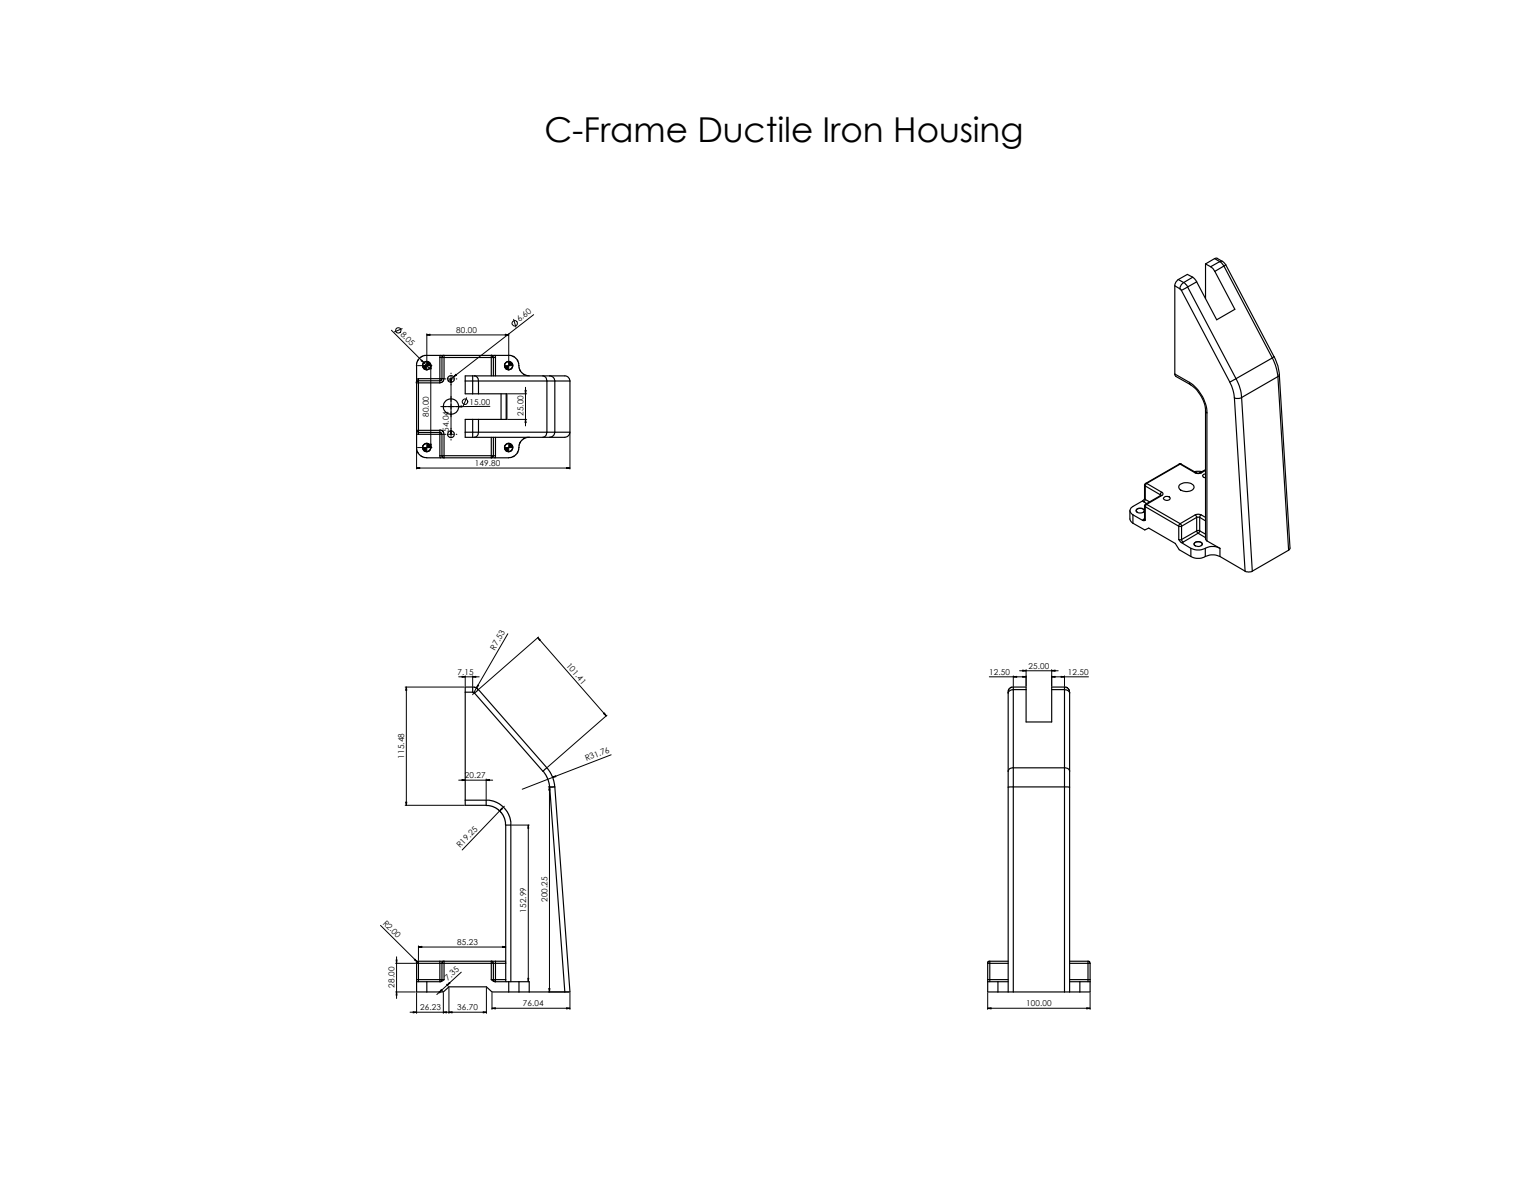
ISO-10303-21;
HEADER;
FILE_DESCRIPTION (('STEP AP214'),
    '1' );
FILE_NAME ('C-Frame Ductile Iron Housing.step',
    '2026-10-20T14:49:59',
    ( '' ),
    ( '' ),
    'SwSTEP 2.0',
    'SolidWorks 2025',
    '' );
FILE_SCHEMA (( 'AUTOMOTIVE_DESIGN' ));
ENDSEC;

DATA;
#1=AXIS2_PLACEMENT_3D ( 'NONE', #1947, #6240, #1422 ) ;
#5=( BOUNDED_CURVE ( )  B_SPLINE_CURVE ( 3, ( #4259, #2824, #7496, #242 ),
 .UNSPECIFIED., .F., .F. ) 
 B_SPLINE_CURVE_WITH_KNOTS ( ( 4, 4 ),
 ( 3.228493165690314637, 4.434806757669079502 ),
 .UNSPECIFIED. ) 
 CURVE ( )  GEOMETRIC_REPRESENTATION_ITEM ( )  RATIONAL_B_SPLINE_CURVE ( ( 1.000000000000000000, 0.8823660295963204891, 0.8823660295963204891, 1.000000000000000000 ) ) 
 REPRESENTATION_ITEM ( '' )  );
#7=EDGE_CURVE ( 'NONE', #389, #4565, #2197, .T. ) ;
#8=VERTEX_POINT ( 'NONE', #6223 ) ;
#15=ORIENTED_EDGE ( 'NONE', *, *, #8479, .F. ) ;
#18=ORIENTED_EDGE ( 'NONE', *, *, #2489, .T. ) ;
#21=DIRECTION ( 'NONE',  ( -1.000000000000000000, 0.000000000000000000, -1.396588258780021135E-16 ) ) ;
#25=DIRECTION ( 'NONE',  ( -1.000000000000000000, 0.000000000000000000, 0.000000000000000000 ) ) ;
#30=ADVANCED_FACE ( 'NONE', ( #9249 ), #6112, .F. ) ;
#31=EDGE_CURVE ( 'NONE', #2894, #7105, #9463, .T. ) ;
#36=VERTEX_POINT ( 'NONE', #6165 ) ;
#37=CIRCLE ( 'NONE', #7311, 10.00000000000000178 ) ;
#40=CARTESIAN_POINT ( 'NONE',  ( 2.108096605167895612E-14, -117.1457019118819005, -25.15769640663941686 ) ) ;
#42=CARTESIAN_POINT ( 'NONE',  ( 39.99999999999998579, -135.1707019118818778, -36.00000000000002842 ) ) ;
#43=DIRECTION ( 'NONE',  ( -1.000000000000000000, 0.000000000000000000, 0.000000000000000000 ) ) ;
#44=LINE ( 'NONE', #8251, #3603 ) ;
#45=VECTOR ( 'NONE', #8925, 1000.000000000000000 ) ;
#46=EDGE_CURVE ( 'NONE', #9808, #836, #8928, .T. ) ;
#47=VERTEX_POINT ( 'NONE', #6006 ) ;
#48=CARTESIAN_POINT ( 'NONE',  ( -16.29350689640809691, -186.9457019118818835, 23.72119897386845722 ) ) ;
#49=ORIENTED_EDGE ( 'NONE', *, *, #1262, .T. ) ;
#55=DIRECTION ( 'NONE',  ( -0.7367503238654704578, -0.6761648913424330720, -0.000000000000000000 ) ) ;
#56=CARTESIAN_POINT ( 'NONE',  ( 99.80027788547049283, -145.1457019118819574, 25.00000000000000000 ) ) ;
#57=LINE ( 'NONE', #8266, #434 ) ;
#58=ORIENTED_EDGE ( 'NONE', *, *, #5513, .T. ) ;
#59=VERTEX_POINT ( 'NONE', #6862 ) ;
#64=ADVANCED_FACE ( 'NONE', ( #10099 ), #3860, .F. ) ;
#65=DIRECTION ( 'NONE',  ( -0.000000000000000000, -0.000000000000000000, -1.000000000000000000 ) ) ;
#69=ORIENTED_EDGE ( 'NONE', *, *, #7396, .F. ) ;
#70=FACE_OUTER_BOUND ( 'NONE', #3100, .T. ) ;
#71=VECTOR ( 'NONE', #3438, 1000.000000000000000 ) ;
#73=CIRCLE ( 'NONE', #8358, 4.025000000000000355 ) ;
#74=ORIENTED_EDGE ( 'NONE', *, *, #80, .F. ) ;
#75=UNCERTAINTY_MEASURE_WITH_UNIT (LENGTH_MEASURE( 1.000000000000000082E-05 ), #6894, 'distance_accuracy_value', 'NONE');
#76=ORIENTED_EDGE ( 'NONE', *, *, #6234, .T. ) ;
#79=LINE ( 'NONE', #3304, #8495 ) ;
#80=EDGE_CURVE ( 'NONE', #1253, #6094, #1141, .T. ) ;
#81=DIRECTION ( 'NONE',  ( 0.000000000000000000, 1.000000000000000000, 0.000000000000000000 ) ) ;
#82=LINE ( 'NONE', #7283, #1628 ) ;
#86=VERTEX_POINT ( 'NONE', #4732 ) ;
#87=CARTESIAN_POINT ( 'NONE',  ( 37.22511195853866894, 17.84145331825995484, -25.00000000000000355 ) ) ;
#92=AXIS2_PLACEMENT_3D ( 'NONE', #1690, #1849, #8953 ) ;
#93=DIRECTION ( 'NONE',  ( 0.000000000000000000, -0.000000000000000000, -1.000000000000000000 ) ) ;
#98=LINE ( 'NONE', #6716, #4014 ) ;
#102=CYLINDRICAL_SURFACE ( 'NONE', #1212, 2.000000000000001776 ) ;
#103=EDGE_CURVE ( 'NONE', #7113, #7038, #645, .T. ) ;
#108=DIRECTION ( 'NONE',  ( 1.000000000000000000, 0.000000000000000000, 0.000000000000000000 ) ) ;
#109=VERTEX_POINT ( 'NONE', #7181 ) ;
#110=ORIENTED_EDGE ( 'NONE', *, *, #8315, .T. ) ;
#111=ORIENTED_EDGE ( 'NONE', *, *, #371, .T. ) ;
#114=ORIENTED_EDGE ( 'NONE', *, *, #3993, .T. ) ;
#115=ORIENTED_EDGE ( 'NONE', *, *, #7748, .F. ) ;
#116=DIRECTION ( 'NONE',  ( 0.000000000000000000, 0.000000000000000000, 1.000000000000000000 ) ) ;
#118=EDGE_CURVE ( 'NONE', #991, #7873, #6383, .T. ) ;
#119=DIRECTION ( 'NONE',  ( -0.000000000000000000, 1.000000000000000000, -0.000000000000000000 ) ) ;
#120=DIRECTION ( 'NONE',  ( -0.000000000000000000, 1.000000000000000000, -0.000000000000000000 ) ) ;
#123=DIRECTION ( 'NONE',  ( -0.000000000000000000, 1.000000000000000000, -0.000000000000000000 ) ) ;
#126=VECTOR ( 'NONE', #3375, 1000.000000000000000 ) ;
#127=CARTESIAN_POINT ( 'NONE',  ( 39.99999999999998579, -115.1457019118818863, -50.00000000000002132 ) ) ;
#128=EDGE_CURVE ( 'NONE', #9477, #9534, #1310, .T. ) ;
#129=VECTOR ( 'NONE', #2614, 1000.000000000000000 ) ;
#130=ORIENTED_EDGE ( 'NONE', *, *, #2088, .F. ) ;
#135=DIRECTION ( 'NONE',  ( 0.000000000000000000, 0.000000000000000000, -1.000000000000000000 ) ) ;
#137=DIRECTION ( 'NONE',  ( 0.000000000000000000, 0.000000000000000000, 1.000000000000000000 ) ) ;
#139=VECTOR ( 'NONE', #10142, 1000.000000000000000 ) ;
#142=EDGE_CURVE ( 'NONE', #5755, #3381, #6273, .T. ) ;
#143=ORIENTED_EDGE ( 'NONE', *, *, #3330, .T. ) ;
#144=DIRECTION ( 'NONE',  ( -1.000000000000000000, 0.000000000000000000, 0.000000000000000000 ) ) ;
#145=ORIENTED_EDGE ( 'NONE', *, *, #5104, .T. ) ;
#149=AXIS2_PLACEMENT_3D ( 'NONE', #5640, #2363, #7980 ) ;
#150=FACE_BOUND ( 'NONE', #8598, .T. ) ;
#151=FACE_OUTER_BOUND ( 'NONE', #4068, .T. ) ;
#159=ORIENTED_EDGE ( 'NONE', *, *, #5597, .F. ) ;
#160=CARTESIAN_POINT ( 'NONE',  ( -2.293506896408097795, 120.5696653505793705, 16.00000000000000711 ) ) ;
#161=FACE_OUTER_BOUND ( 'NONE', #8002, .T. ) ;
#162=DIRECTION ( 'NONE',  ( 0.000000000000000000, 0.000000000000000000, -1.000000000000000000 ) ) ;
#163=CARTESIAN_POINT ( 'NONE',  ( 0.000000000000000000, -135.1457019118818721, 49.99999999999997868 ) ) ;
#164=DIRECTION ( 'NONE',  ( -0.000000000000000000, 1.000000000000000000, -0.000000000000000000 ) ) ;
#165=DIRECTION ( 'NONE',  ( 1.000000000000000000, 0.000000000000000000, -0.000000000000000000 ) ) ;
#170=EDGE_LOOP ( 'NONE', ( #1521, #9934, #3722, #2301 ) ) ;
#172=VERTEX_POINT ( 'NONE', #5530 ) ;
#174=CARTESIAN_POINT ( 'NONE',  ( 4.856471286862176662, 145.0444252872335937, -25.00000000000000355 ) ) ;
#175=CARTESIAN_POINT ( 'NONE',  ( 39.99999999999998579, -135.1707019118818778, -40.00000000000002132 ) ) ;
#176=ORIENTED_EDGE ( 'NONE', *, *, #2184, .F. ) ;
#178=ORIENTED_EDGE ( 'NONE', *, *, #10204, .T. ) ;
#180=ADVANCED_FACE ( 'NONE', ( #7280 ), #10317, .T. ) ;
#181=ORIENTED_EDGE ( 'NONE', *, *, #259, .T. ) ;
#184=DIRECTION ( 'NONE',  ( 0.6761648913424331830, 0.7367503238654705688, 0.000000000000000000 ) ) ;
#185=FACE_OUTER_BOUND ( 'NONE', #1495, .T. ) ;
#189=ORIENTED_EDGE ( 'NONE', *, *, #3670, .T. ) ;
#192=PRODUCT_CONTEXT ( 'NONE', #5163, 'mechanical' ) ;
#193=ORIENTED_EDGE ( 'NONE', *, *, #118, .T. ) ;
#194=CARTESIAN_POINT ( 'NONE',  ( 0.000000000000000000, -135.1457019118818721, 0.000000000000000000 ) ) ;
#196=ADVANCED_FACE ( 'NONE', ( #3094 ), #2303, .F. ) ;
#201=DIRECTION ( 'NONE',  ( -0.000000000000000000, 1.000000000000000000, -0.000000000000000000 ) ) ;
#204=AXIS2_PLACEMENT_3D ( 'NONE', #9863, #838, #6454 ) ;
#206=CIRCLE ( 'NONE', #9340, 5.000000000000000888 ) ;
#207=EDGE_LOOP ( 'NONE', ( #1735, #9870, #2298, #4217 ) ) ;
#208=DIRECTION ( 'NONE',  ( -0.000000000000000000, -0.000000000000000000, -1.000000000000000000 ) ) ;
#210=DIRECTION ( 'NONE',  ( 0.000000000000000000, -1.000000000000000000, 0.000000000000000000 ) ) ;
#211=DIRECTION ( 'NONE',  ( 1.000000000000000000, 0.000000000000000000, 0.000000000000000000 ) ) ;
#215=CARTESIAN_POINT ( 'NONE',  ( 39.99999999999997158, -135.1707019118818778, 35.99999999999998579 ) ) ;
#216=ORIENTED_EDGE ( 'NONE', *, *, #1932, .F. ) ;
#219=ORIENTED_EDGE ( 'NONE', *, *, #8508, .T. ) ;
#220=CIRCLE ( 'NONE', #5954, 2.000000000000001776 ) ;
#222=DIRECTION ( 'NONE',  ( 1.000000000000000000, -0.000000000000000000, -0.000000000000000000 ) ) ;
#223=ADVANCED_FACE ( 'NONE', ( #968 ), #9262, .F. ) ;
#225=EDGE_CURVE ( 'NONE', #5542, #7357, #9074, .T. ) ;
#226=ORIENTED_EDGE ( 'NONE', *, *, #6379, .T. ) ;
#227=CARTESIAN_POINT ( 'NONE',  ( 14.70649310359190309, 120.5696653505793705, 20.00000000000000711 ) ) ;
#228=TOROIDAL_SURFACE ( 'NONE', #6479, 2.525240063345735475, 5.000000000000000000 ) ;
#230=CARTESIAN_POINT ( 'NONE',  ( 14.70649310359190309, 120.5696653505793705, 20.00000000000000711 ) ) ;
#232=ORIENTED_EDGE ( 'NONE', *, *, #10101, .T. ) ;
#234=CARTESIAN_POINT ( 'NONE',  ( -40.00000000000001421, -145.1457019118819005, -40.00000000000002132 ) ) ;
#235=VECTOR ( 'NONE', #6566, 1000.000000000000000 ) ;
#239=EDGE_CURVE ( 'NONE', #4318, #3843, #3408, .T. ) ;
#242=CARTESIAN_POINT ( 'NONE',  ( -18.34874108452141783, -140.1746510883711778, 7.212905963064383918 ) ) ;
#243=ORIENTED_EDGE ( 'NONE', *, *, #6508, .F. ) ;
#244=CARTESIAN_POINT ( 'NONE',  ( -40.00000000000002842, -135.1457019118818721, 39.99999999999997868 ) ) ;
#246=ORIENTED_EDGE ( 'NONE', *, *, #9487, .F. ) ;
#248=LINE ( 'NONE', #2462, #7946 ) ;
#249=VERTEX_POINT ( 'NONE', #5785 ) ;
#251=EDGE_CURVE ( 'NONE', #7304, #5030, #3169, .T. ) ;
#252=FACE_BOUND ( 'NONE', #5488, .T. ) ;
#253=CARTESIAN_POINT ( 'NONE',  ( -50.00000000000002132, -115.1457019118818863, 23.15769640663938134 ) ) ;
#256=DIRECTION ( 'NONE',  ( 0.000000000000000000, 0.000000000000000000, -1.000000000000000000 ) ) ;
#257=CARTESIAN_POINT ( 'NONE',  ( -23.15769640663940976, -133.1457019118818721, 49.99999999999997868 ) ) ;
#259=EDGE_CURVE ( 'NONE', #9948, #541, #8974, .T. ) ;
#260=EDGE_LOOP ( 'NONE', ( #7752, #8876, #7839, #4575 ) ) ;
#261=AXIS2_PLACEMENT_3D ( 'NONE', #3282, #9005, #108 ) ;
#262=DIRECTION ( 'NONE',  ( 1.000000000000000000, 0.000000000000000000, 0.000000000000000000 ) ) ;
#265=FACE_OUTER_BOUND ( 'NONE', #5639, .T. ) ;
#266=DIRECTION ( 'NONE',  ( -0.000000000000000000, 1.000000000000000000, -0.000000000000000000 ) ) ;
#267=B_SPLINE_CURVE_WITH_KNOTS ( 'NONE', 3,
 ( #1751, #6037, #5296, #7584 ),
 .UNSPECIFIED., .F., .F.,
 ( 4, 4 ),
 ( 0.000000000000000000, 0.0007942240325546930492 ),
 .UNSPECIFIED. ) ;
#269=DIRECTION ( 'NONE',  ( 0.000000000000000000, 0.000000000000000000, -1.000000000000000000 ) ) ;
#271=CIRCLE ( 'NONE', #8898, 4.999999999999997335 ) ;
#273=ORIENTED_EDGE ( 'NONE', *, *, #8937, .T. ) ;
#275=ORIENTED_EDGE ( 'NONE', *, *, #9151, .T. ) ;
#280=ORIENTED_EDGE ( 'NONE', *, *, #3281, .F. ) ;
#282=AXIS2_PLACEMENT_3D ( 'NONE', #1944, #4741, #724 ) ;
#284=CYLINDRICAL_SURFACE ( 'NONE', #9989, 2.000000000000001776 ) ;
#285=CIRCLE ( 'NONE', #7057, 3.999999999999996447 ) ;
#287=EDGE_CURVE ( 'NONE', #249, #2514, #5099, .T. ) ;
#293=CARTESIAN_POINT ( 'NONE',  ( -48.00000000000002132, -133.1457019118818721, -27.15769640663945594 ) ) ;
#296=DIRECTION ( 'NONE',  ( -0.000000000000000000, 1.000000000000000000, -0.000000000000000000 ) ) ;
#297=CARTESIAN_POINT ( 'NONE',  ( 39.99999999999997158, -135.1457019118818721, 39.99999999999997868 ) ) ;
#298=ORIENTED_EDGE ( 'NONE', *, *, #6850, .F. ) ;
#301=ORIENTED_EDGE ( 'NONE', *, *, #542, .F. ) ;
#305=AXIS2_PLACEMENT_3D ( 'NONE', #4703, #7939, #5550 ) ;
#309=DIRECTION ( 'NONE',  ( -0.000000000000000000, -0.000000000000000000, 1.000000000000000000 ) ) ;
#311=EDGE_LOOP ( 'NONE', ( #929, #9154, #4963 ) ) ;
#312=AXIS2_PLACEMENT_3D ( 'NONE', #483, #2971, #4458 ) ;
#313=CARTESIAN_POINT ( 'NONE',  ( 53.40242741783141156, 42.08684478514406635, -30.00000000000000355 ) ) ;
#319=ORIENTED_EDGE ( 'NONE', *, *, #618, .T. ) ;
#320=DIRECTION ( 'NONE',  ( -1.387778780781445676E-16, 0.000000000000000000, 1.000000000000000000 ) ) ;
#321=DIRECTION ( 'NONE',  ( 0.000000000000000000, 0.000000000000000000, 1.000000000000000000 ) ) ;
#323=CARTESIAN_POINT ( 'NONE',  ( -38.19229777560033057, 37.08684478514405214, -12.50000000000000000 ) ) ;
#327=ORIENTED_EDGE ( 'NONE', *, *, #7111, .T. ) ;
#329=CARTESIAN_POINT ( 'NONE',  ( 14.70649310359190309, 120.5696653505793705, -20.00000000000000711 ) ) ;
#330=CIRCLE ( 'NONE', #4045, 4.000000000000000000 ) ;
#332=EDGE_CURVE ( 'NONE', #8658, #7935, #9280, .T. ) ;
#335=DIRECTION ( 'NONE',  ( 0.000000000000000000, 0.000000000000000000, 1.000000000000000000 ) ) ;
#336=ORIENTED_EDGE ( 'NONE', *, *, #3079, .T. ) ;
#337=CARTESIAN_POINT ( 'NONE',  ( 14.70649310359190309, 80.56966535057935630, -20.00000000000000711 ) ) ;
#340=ORIENTED_EDGE ( 'NONE', *, *, #1843, .F. ) ;
#346=CARTESIAN_POINT ( 'NONE',  ( 37.22797271129282848, -133.4137847133962396, -25.17122046401099311 ) ) ;
#348=DIRECTION ( 'NONE',  ( 0.000000000000000000, 1.000000000000000000, -0.000000000000000000 ) ) ;
#349=ORIENTED_EDGE ( 'NONE', *, *, #1530, .T. ) ;
#351=CARTESIAN_POINT ( 'NONE',  ( 39.99999999999998579, -135.1457019118818721, -40.00000000000002132 ) ) ;
#352=DIRECTION ( 'NONE',  ( 0.000000000000000000, 0.000000000000000000, 1.000000000000000000 ) ) ;
#359=ORIENTED_EDGE ( 'NONE', *, *, #6276, .F. ) ;
#366=ORIENTED_EDGE ( 'NONE', *, *, #3251, .T. ) ;
#371=EDGE_CURVE ( 'NONE', #6079, #5542, #9235, .T. ) ;
#373=EDGE_CURVE ( 'NONE', #3710, #6945, #2925, .T. ) ;
#375=ORIENTED_EDGE ( 'NONE', *, *, #6294, .F. ) ;
#377=ORIENTED_EDGE ( 'NONE', *, *, #2708, .T. ) ;
#381=LINE ( 'NONE', #2917, #3516 ) ;
#385=AXIS2_PLACEMENT_3D ( 'NONE', #470, #266, #3704 ) ;
#388=ORIENTED_EDGE ( 'NONE', *, *, #4709, .T. ) ;
#389=VERTEX_POINT ( 'NONE', #6099 ) ;
#391=LINE ( 'NONE', #7015, #708 ) ;
#392=DIRECTION ( 'NONE',  ( -0.7525569905852185215, -0.6585271261848818503, 0.000000000000000000 ) ) ;
#400=CARTESIAN_POINT ( 'NONE',  ( 99.80027788547049283, -145.1457019118819005, 25.00000000000000000 ) ) ;
#403=LINE ( 'NONE', #4479, #10289 ) ;
#406=AXIS2_PLACEMENT_3D ( 'NONE', #8418, #9973, #3651 ) ;
#408=CARTESIAN_POINT ( 'NONE',  ( -16.29350689640809691, -140.1746510883711778, -27.01918567566963247 ) ) ;
#412=EDGE_LOOP ( 'NONE', ( #6955, #1615, #901, #8803 ) ) ;
#413=CARTESIAN_POINT ( 'NONE',  ( 39.99999999999997158, -145.1457019118819005, 43.99999999999997158 ) ) ;
#414=EDGE_CURVE ( 'NONE', #7304, #3508, #5358, .T. ) ;
#415=VERTEX_POINT ( 'NONE', #7799 ) ;
#416=AXIS2_PLACEMENT_3D ( 'NONE', #6605, #8136, #2577 ) ;
#421=FACE_OUTER_BOUND ( 'NONE', #4486, .T. ) ;
#424=VECTOR ( 'NONE', #10366, 1000.000000000000000 ) ;
#425=ORIENTED_EDGE ( 'NONE', *, *, #4709, .F. ) ;
#426=VERTEX_POINT ( 'NONE', #6154 ) ;
#427=CARTESIAN_POINT ( 'NONE',  ( 39.99999999999998579, -135.1457019118818721, -40.00000000000002132 ) ) ;
#429=EDGE_CURVE ( 'NONE', #10221, #9616, #9343, .T. ) ;
#433=DIRECTION ( 'NONE',  ( 0.000000000000000000, 0.000000000000000000, 1.000000000000000000 ) ) ;
#434=VECTOR ( 'NONE', #2697, 1000.000000000000000 ) ;
#436=CARTESIAN_POINT ( 'NONE',  ( 39.99999999999998579, -135.1457019118818721, -44.02500000000001990 ) ) ;
#437=CIRCLE ( 'NONE', #6179, 10.00000000000000178 ) ;
#440=ORIENTED_EDGE ( 'NONE', *, *, #2696, .F. ) ;
#446=CYLINDRICAL_SURFACE ( 'NONE', #9247, 1.999999999999998224 ) ;
#448=FACE_OUTER_BOUND ( 'NONE', #668, .T. ) ;
#449=AXIS2_PLACEMENT_3D ( 'NONE', #1185, #3570, #1133 ) ;
#451=DIRECTION ( 'NONE',  ( 1.000000000000000000, 0.000000000000000000, -0.000000000000000000 ) ) ;
#453=DIRECTION ( 'NONE',  ( 8.379529552680108569E-16, 0.000000000000000000, -1.000000000000000000 ) ) ;
#454=ORIENTED_EDGE ( 'NONE', *, *, #516, .F. ) ;
#456=CARTESIAN_POINT ( 'NONE',  ( 23.15769640663935292, -117.1457019118819005, 2.263923683133336310E-14 ) ) ;
#457=EDGE_CURVE ( 'NONE', #10082, #9303, #1997, .T. ) ;
#461=ORIENTED_EDGE ( 'NONE', *, *, #1064, .F. ) ;
#462=CARTESIAN_POINT ( 'NONE',  ( 0.000000000000000000, -135.1457019118818721, -30.00000000000000355 ) ) ;
#463=AXIS2_PLACEMENT_3D ( 'NONE', #984, #7454, #8830 ) ;
#464=ORIENTED_EDGE ( 'NONE', *, *, #46, .F. ) ;
#465=CARTESIAN_POINT ( 'NONE',  ( -23.15769640663937423, -117.1457019118819005, -50.00000000000002132 ) ) ;
#470=CARTESIAN_POINT ( 'NONE',  ( 39.99999999999997158, -135.1457019118818721, 39.99999999999997868 ) ) ;
#473=DIRECTION ( 'NONE',  ( -0.000000000000000000, -1.000000000000000000, -0.000000000000000000 ) ) ;
#475=EDGE_CURVE ( 'NONE', #3710, #4318, #8599, .T. ) ;
#478=CARTESIAN_POINT ( 'NONE',  ( -2.293506896408094242, 152.5696653505793279, -12.50000000000000000 ) ) ;
#480=CARTESIAN_POINT ( 'NONE',  ( 14.70649310359190309, 120.5696653505793705, 20.00000000000000711 ) ) ;
#482=CARTESIAN_POINT ( 'NONE',  ( 38.19229777560031636, 118.3760186273086816, -12.50000000000000000 ) ) ;
#483=CARTESIAN_POINT ( 'NONE',  ( 0.000000000000000000, -115.1457019118818863, -50.00000000000002132 ) ) ;
#485=AXIS2_PLACEMENT_3D ( 'NONE', #1777, #6653, #7502 ) ;
#492=ORIENTED_EDGE ( 'NONE', *, *, #6447, .F. ) ;
#496=DIRECTION ( 'NONE',  ( 0.000000000000000000, 1.000000000000000000, 0.000000000000000000 ) ) ;
#499=LINE ( 'NONE', #10311, #7721 ) ;
#500=EDGE_CURVE ( 'NONE', #47, #3843, #7698, .T. ) ;
#505=CARTESIAN_POINT ( 'NONE',  ( 25.15769640663936002, -115.1457019118818863, -3.513494341946486113E-15 ) ) ;
#507=DIRECTION ( 'NONE',  ( -1.000000000000000000, 0.000000000000000000, 0.000000000000000000 ) ) ;
#508=DIRECTION ( 'NONE',  ( -0.000000000000000000, 1.000000000000000000, -0.000000000000000000 ) ) ;
#511=CYLINDRICAL_SURFACE ( 'NONE', #5792, 4.999999999999997335 ) ;
#514=LINE ( 'NONE', #8516, #2322 ) ;
#515=ORIENTED_EDGE ( 'NONE', *, *, #6735, .T. ) ;
#516=EDGE_CURVE ( 'NONE', #9939, #3381, #7904, .T. ) ;
#520=( LENGTH_UNIT ( ) NAMED_UNIT ( * ) SI_UNIT ( .MILLI., .METRE. ) );
#521=DIRECTION ( 'NONE',  ( 0.000000000000000000, -1.000000000000000000, 0.000000000000000000 ) ) ;
#523=DIRECTION ( 'NONE',  ( 0.000000000000000000, 1.000000000000000000, -0.000000000000000000 ) ) ;
#527=AXIS2_PLACEMENT_3D ( 'NONE', #7457, #1037, #6552 ) ;
#528=ORIENTED_EDGE ( 'NONE', *, *, #8703, .F. ) ;
#529=ADVANCED_FACE ( 'NONE', ( #748 ), #598, .F. ) ;
#530=DIRECTION ( 'NONE',  ( -1.387778780781445676E-16, 0.000000000000000000, 1.000000000000000000 ) ) ;
#531=CARTESIAN_POINT ( 'NONE',  ( -2.293506896408097795, 152.5696653505793279, 30.00000000000000355 ) ) ;
#533=LINE ( 'NONE', #2178, #8761 ) ;
#535=VECTOR ( 'NONE', #5204, 1000.000000000000227 ) ;
#538=AXIS2_PLACEMENT_3D ( 'NONE', #3174, #3070, #8843 ) ;
#539=ORIENTED_EDGE ( 'NONE', *, *, #7426, .F. ) ;
#540=AXIS2_PLACEMENT_3D ( 'NONE', #9014, #1857, #5669 ) ;
#541=VERTEX_POINT ( 'NONE', #3185 ) ;
#542=EDGE_CURVE ( 'NONE', #1314, #8114, #798, .T. ) ;
#546=FACE_OUTER_BOUND ( 'NONE', #2266, .T. ) ;
#547=DIRECTION ( 'NONE',  ( -0.000000000000000000, 1.000000000000000000, -0.000000000000000000 ) ) ;
#548=DIRECTION ( 'NONE',  ( 0.000000000000000000, -0.000000000000000000, -1.000000000000000000 ) ) ;
#549=AXIS2_PLACEMENT_3D ( 'NONE', #9186, #9892, #1766 ) ;
#550=ORIENTED_EDGE ( 'NONE', *, *, #3594, .F. ) ;
#552=CARTESIAN_POINT ( 'NONE',  ( -48.00000000000002132, -117.1457019118819005, -25.15769640663945950 ) ) ;
#553=DIRECTION ( 'NONE',  ( 1.000000000000000000, 0.000000000000000000, 0.000000000000000000 ) ) ;
#554=EDGE_CURVE ( 'NONE', #10372, #47, #7122, .T. ) ;
#555=ORIENTED_EDGE ( 'NONE', *, *, #457, .T. ) ;
#557=CIRCLE ( 'NONE', #1228, 2.000000000000001776 ) ;
#560=CARTESIAN_POINT ( 'NONE',  ( 25.93999053166053415, -135.0799163051958942, -50.00000000000002132 ) ) ;
#561=CARTESIAN_POINT ( 'NONE',  ( -50.00000000000001421, -145.1457019118819005, -40.00000000000002132 ) ) ;
#563=DIRECTION ( 'NONE',  ( -1.000000000000000000, 0.000000000000000000, 0.000000000000000000 ) ) ;
#564=AXIS2_PLACEMENT_3D ( 'NONE', #9552, #1379, #738 ) ;
#568=CARTESIAN_POINT ( 'NONE',  ( -40.00000000000002842, -135.1457019118818721, 39.99999999999997868 ) ) ;
#569=ORIENTED_EDGE ( 'NONE', *, *, #2486, .T. ) ;
#570=ADVANCED_FACE ( 'NONE', ( #6415 ), #698, .F. ) ;
#573=DIRECTION ( 'NONE',  ( 0.000000000000000000, 1.000000000000000000, 0.000000000000000000 ) ) ;
#574=AXIS2_PLACEMENT_3D ( 'NONE', #10123, #6882, #3549 ) ;
#575=LINE ( 'NONE', #9043, #126 ) ;
#578=FACE_BOUND ( 'NONE', #834, .T. ) ;
#580=ADVANCED_FACE ( 'NONE', ( #5467, #8756 ), #7961, .F. ) ;
#581=VERTEX_POINT ( 'NONE', #8700 ) ;
#583=DIRECTION ( 'NONE',  ( 0.000000000000000000, 0.000000000000000000, -1.000000000000000000 ) ) ;
#586=CARTESIAN_POINT ( 'NONE',  ( -48.00000000000002132, -117.1457019118819005, -23.15769640663945594 ) ) ;
#587=DIRECTION ( 'NONE',  ( -0.000000000000000000, 0.000000000000000000, -1.000000000000000000 ) ) ;
#589=CARTESIAN_POINT ( 'NONE',  ( 14.70649310359190309, 120.5696653505793705, -20.00000000000000711 ) ) ;
#595=CIRCLE ( 'NONE', #4810, 2.000000000000001776 ) ;
#598=PLANE ( 'NONE',  #1493 ) ;
#599=CARTESIAN_POINT ( 'NONE',  ( 42.22511195853869026, -135.1457019118818721, -25.00000000000000355 ) ) ;
#602=DIRECTION ( 'NONE',  ( -0.000000000000000000, 1.000000000000000000, -0.000000000000000000 ) ) ;
#609=AXIS2_PLACEMENT_3D ( 'NONE', #4481, #3581, #5958 ) ;
#611=CARTESIAN_POINT ( 'NONE',  ( 25.28853996896956247, -134.8487302617674857, -50.00000000000001421 ) ) ;
#612=DIRECTION ( 'NONE',  ( 1.000000000000000000, 0.000000000000000000, 1.387778780781445676E-16 ) ) ;
#616=ADVANCED_FACE ( 'NONE', ( #8805 ), #1548, .T. ) ;
#618=EDGE_CURVE ( 'NONE', #5017, #8294, #9061, .T. ) ;
#619=ORIENTED_EDGE ( 'NONE', *, *, #4744, .F. ) ;
#620=CIRCLE ( 'NONE', #8401, 2.000000000000001776 ) ;
#626=CIRCLE ( 'NONE', #3497, 2.000000000000001776 ) ;
#627=DIRECTION ( 'NONE',  ( -0.000000000000000000, 1.000000000000000000, -0.000000000000000000 ) ) ;
#628=CARTESIAN_POINT ( 'NONE',  ( 39.99999999999998579, -135.1457019118818721, -40.00000000000002132 ) ) ;
#629=DIRECTION ( 'NONE',  ( -0.000000000000000000, 1.000000000000000000, -0.000000000000000000 ) ) ;
#631=PLANE ( 'NONE',  #5090 ) ;
#635=ORIENTED_EDGE ( 'NONE', *, *, #3138, .T. ) ;
#636=VECTOR ( 'NONE', #2330, 1000.000000000000000 ) ;
#637=CARTESIAN_POINT ( 'NONE',  ( 4.856471286862175774, 152.5696653505793279, -25.00000000000000355 ) ) ;
#638=ADVANCED_BREP_SHAPE_REPRESENTATION ( '', ( #3440, #4601 ), #9171 ) ;
#639=VECTOR ( 'NONE', #7530, 1000.000000000000000 ) ;
#640=VERTEX_POINT ( 'NONE', #4082 ) ;
#641=CARTESIAN_POINT ( 'NONE',  ( -16.29350689640809691, -140.1746510883711778, 0.000000000000000000 ) ) ;
#643=FACE_OUTER_BOUND ( 'NONE', #4818, .T. ) ;
#644=FACE_OUTER_BOUND ( 'NONE', #7569, .T. ) ;
#645=CIRCLE ( 'NONE', #4022, 2.000000000000001776 ) ;
#648=ORIENTED_EDGE ( 'NONE', *, *, #9261, .F. ) ;
#649=ORIENTED_EDGE ( 'NONE', *, *, #8829, .F. ) ;
#650=CIRCLE ( 'NONE', #9099, 5.000000000000000888 ) ;
#653=ORIENTED_EDGE ( 'NONE', *, *, #2945, .T. ) ;
#655=EDGE_CURVE ( 'NONE', #2542, #4089, #1011, .T. ) ;
#659=DIRECTION ( 'NONE',  ( 0.000000000000000000, 0.000000000000000000, -1.000000000000000000 ) ) ;
#663=ORIENTED_EDGE ( 'NONE', *, *, #7153, .F. ) ;
#666=CARTESIAN_POINT ( 'NONE',  ( 39.99999999999998579, -145.1457019118819005, -36.00000000000002842 ) ) ;
#668=EDGE_LOOP ( 'NONE', ( #1329, #7723 ) ) ;
#669=CARTESIAN_POINT ( 'NONE',  ( -16.29350689640809691, -186.9457019118818835, 0.000000000000000000 ) ) ;
#671=ORIENTED_EDGE ( 'NONE', *, *, #4878, .T. ) ;
#681=FACE_OUTER_BOUND ( 'NONE', #5766, .T. ) ;
#683=DIRECTION ( 'NONE',  ( 0.000000000000000000, 0.000000000000000000, 1.000000000000000000 ) ) ;
#685=DIRECTION ( 'NONE',  ( 1.000000000000000000, 0.000000000000000000, 0.000000000000000000 ) ) ;
#688=CARTESIAN_POINT ( 'NONE',  ( -25.15769640663940976, -133.1457019118818721, 47.99999999999997868 ) ) ;
#693=PLANE ( 'NONE',  #3300 ) ;
#694=DIRECTION ( 'NONE',  ( 0.000000000000000000, -1.000000000000000000, 0.000000000000000000 ) ) ;
#695=ORIENTED_EDGE ( 'NONE', *, *, #3251, .F. ) ;
#696=EDGE_LOOP ( 'NONE', ( #7582, #6873 ) ) ;
#698=CYLINDRICAL_SURFACE ( 'NONE', #3691, 3.297986701801175258 ) ;
#700=AXIS2_PLACEMENT_3D ( 'NONE', #4653, #4706, #8680 ) ;
#701=LINE ( 'NONE', #5621, #2314 ) ;
#704=ORIENTED_EDGE ( 'NONE', *, *, #31, .F. ) ;
#705=DIRECTION ( 'NONE',  ( -1.000000000000000000, 0.000000000000000000, 0.000000000000000000 ) ) ;
#707=CIRCLE ( 'NONE', #1387, 19.24539146688411506 ) ;
#708=VECTOR ( 'NONE', #5359, 1000.000000000000000 ) ;
#710=CARTESIAN_POINT ( 'NONE',  ( 27.15769640663935647, -133.1457019118818721, 2.654968395591742513E-14 ) ) ;
#713=AXIS2_PLACEMENT_3D ( 'NONE', #6468, #8162, #5720 ) ;
#714=CARTESIAN_POINT ( 'NONE',  ( 26.62179802177715615, -135.1457019118818721, -50.00000000000002132 ) ) ;
#717=CARTESIAN_POINT ( 'NONE',  ( -25.15769640663939199, -133.1457019118818721, -27.15769640663944173 ) ) ;
#720=CIRCLE ( 'NONE', #9019, 4.000000000000000000 ) ;
#721=LINE ( 'NONE', #3910, #10314 ) ;
#724=DIRECTION ( 'NONE',  ( 0.000000000000000000, 0.000000000000000000, -1.000000000000000000 ) ) ;
#726=DIRECTION ( 'NONE',  ( -0.000000000000000000, 1.000000000000000000, -0.000000000000000000 ) ) ;
#730=DIRECTION ( 'NONE',  ( -9.776117811460147207E-16, 0.000000000000000000, 1.000000000000000000 ) ) ;
#732=VERTEX_POINT ( 'NONE', #2652 ) ;
#733=CARTESIAN_POINT ( 'NONE',  ( 38.19229777560031636, -43.28483205141633761, 12.50000000000000000 ) ) ;
#738=DIRECTION ( 'NONE',  ( 0.000000000000000000, -0.000000000000000000, 1.000000000000000000 ) ) ;
#742=AXIS2_PLACEMENT_3D ( 'NONE', #6990, #7887, #1423 ) ;
#743=ORIENTED_EDGE ( 'NONE', *, *, #2625, .F. ) ;
#746=EDGE_CURVE ( 'NONE', #4432, #1005, #6398, .T. ) ;
#747=ORIENTED_EDGE ( 'NONE', *, *, #7309, .T. ) ;
#748=FACE_OUTER_BOUND ( 'NONE', #1862, .T. ) ;
#751=CARTESIAN_POINT ( 'NONE',  ( 14.70649310359190309, 120.5696653505793705, -24.00000000000000711 ) ) ;
#752=CARTESIAN_POINT ( 'NONE',  ( 25.15769640663936357, -133.1457019118818721, 27.15769640663938489 ) ) ;
#754=ORIENTED_EDGE ( 'NONE', *, *, #8274, .T. ) ;
#757=EDGE_CURVE ( 'NONE', #6846, #5066, #8265, .T. ) ;
#760=CARTESIAN_POINT ( 'NONE',  ( 23.15769640663936713, -117.1457019118819005, 47.99999999999997868 ) ) ;
#762=DIRECTION ( 'NONE',  ( -0.000000000000000000, 1.000000000000000000, 0.000000000000000000 ) ) ;
#764=ORIENTED_EDGE ( 'NONE', *, *, #7097, .F. ) ;
#766=ORIENTED_EDGE ( 'NONE', *, *, #6509, .F. ) ;
#770=APPLICATION_CONTEXT ( 'automotive_design' ) ;
#771=ORIENTED_EDGE ( 'NONE', *, *, #2304, .T. ) ;
#773=FACE_OUTER_BOUND ( 'NONE', #6412, .T. ) ;
#774=LINE ( 'NONE', #5749, #5140 ) ;
#775=CARTESIAN_POINT ( 'NONE',  ( -27.15769640663940621, -133.1457019118818721, -3.792811993702496405E-15 ) ) ;
#776=CIRCLE ( 'NONE', #10093, 10.00000000000000178 ) ;
#786=DIRECTION ( 'NONE',  ( 0.000000000000000000, 0.000000000000000000, -1.000000000000000000 ) ) ;
#790=CYLINDRICAL_SURFACE ( 'NONE', #7011, 4.000000000000000000 ) ;
#791=DIRECTION ( 'NONE',  ( 0.000000000000000000, 0.000000000000000000, -1.000000000000000000 ) ) ;
#795=AXIS2_PLACEMENT_3D ( 'NONE', #9143, #5116, #4324 ) ;
#796=EDGE_LOOP ( 'NONE', ( #3033, #3285, #2044, #4290, #4720, #6254, #6792, #181, #8225, #1496, #6918, #653, #4433, #3564, #275, #5135 ) ) ;
#798=LINE ( 'NONE', #7169, #6391 ) ;
#800=AXIS2_PLACEMENT_3D ( 'NONE', #1242, #3197, #6426 ) ;
#803=EDGE_CURVE ( 'NONE', #1658, #1518, #5219, .T. ) ;
#806=VECTOR ( 'NONE', #507, 1000.000000000000000 ) ;
#809=ORIENTED_EDGE ( 'NONE', *, *, #9423, .T. ) ;
#813=ORIENTED_EDGE ( 'NONE', *, *, #3298, .T. ) ;
#815=DIRECTION ( 'NONE',  ( 0.000000000000000000, 0.000000000000000000, -1.000000000000000000 ) ) ;
#816=VECTOR ( 'NONE', #7358, 1000.000000000000000 ) ;
#817=EDGE_CURVE ( 'NONE', #4776, #9808, #8534, .T. ) ;
#818=FACE_OUTER_BOUND ( 'NONE', #3605, .T. ) ;
#819=CARTESIAN_POINT ( 'NONE',  ( 37.25478555609232245, -134.3993646471907084, -25.57704176894851855 ) ) ;
#820=ORIENTED_EDGE ( 'NONE', *, *, #10303, .T. ) ;
#823=CARTESIAN_POINT ( 'NONE',  ( 4.856471286862173997, 152.5696653505793279, 12.50000000000000000 ) ) ;
#824=ORIENTED_EDGE ( 'NONE', *, *, #3937, .F. ) ;
#825=AXIS2_PLACEMENT_3D ( 'NONE', #194, #4265, #2629 ) ;
#826=VERTEX_POINT ( 'NONE', #2700 ) ;
#829=DIRECTION ( 'NONE',  ( 0.000000000000000000, 0.000000000000000000, -1.000000000000000000 ) ) ;
#830=FACE_OUTER_BOUND ( 'NONE', #1137, .T. ) ;
#834=EDGE_LOOP ( 'NONE', ( #2251, #3043 ) ) ;
#835=DIRECTION ( 'NONE',  ( 0.000000000000000000, 0.000000000000000000, 1.000000000000000000 ) ) ;
#836=VERTEX_POINT ( 'NONE', #2012 ) ;
#837=CARTESIAN_POINT ( 'NONE',  ( -16.29350689640809691, -186.9457019118818835, -23.72119897386845722 ) ) ;
#838=DIRECTION ( 'NONE',  ( -1.000000000000000000, 0.000000000000000000, 0.000000000000000000 ) ) ;
#839=DIRECTION ( 'NONE',  ( -0.000000000000000000, 1.000000000000000000, -0.000000000000000000 ) ) ;
#842=DIRECTION ( 'NONE',  ( 0.6585271261848804070, -0.7525569905852197428, 0.000000000000000000 ) ) ;
#844=ORIENTED_EDGE ( 'NONE', *, *, #4744, .T. ) ;
#847=VERTEX_POINT ( 'NONE', #6947 ) ;
#857=ADVANCED_FACE ( 'NONE', ( #3501 ), #7687, .F. ) ;
#862=CARTESIAN_POINT ( 'NONE',  ( 39.99999999999998579, -145.1457019118819005, -50.00000000000002132 ) ) ;
#863=DIRECTION ( 'NONE',  ( 0.000000000000000000, -1.000000000000000000, 0.000000000000000000 ) ) ;
#864=AXIS2_PLACEMENT_3D ( 'NONE', #244, #3308, #4941 ) ;
#865=EDGE_LOOP ( 'NONE', ( #454, #7854, #1982, #1701 ) ) ;
#867=DIRECTION ( 'NONE',  ( 0.000000000000000000, 0.000000000000000000, 1.000000000000000000 ) ) ;
#869=VERTEX_POINT ( 'NONE', #5345 ) ;
#870=ADVANCED_FACE ( 'NONE', ( #10077 ), #8372, .T. ) ;
#871=EDGE_CURVE ( 'NONE', #4076, #4046, #1907, .T. ) ;
#872=CARTESIAN_POINT ( 'NONE',  ( -26.62179802177716326, -135.1457019118818721, 49.99999999999997868 ) ) ;
#873=ORIENTED_EDGE ( 'NONE', *, *, #4154, .F. ) ;
#874=AXIS2_PLACEMENT_3D ( 'NONE', #5517, #1500, #7271 ) ;
#876=CARTESIAN_POINT ( 'NONE',  ( -23.15769640663940976, -133.1457019118818721, 47.99999999999997868 ) ) ;
#881=CIRCLE ( 'NONE', #385, 4.025000000000000355 ) ;
#882=CIRCLE ( 'NONE', #9179, 3.999999999999989786 ) ;
#883=ORIENTED_EDGE ( 'NONE', *, *, #5880, .F. ) ;
#890=DIRECTION ( 'NONE',  ( 1.000000000000000000, 0.000000000000000000, 0.000000000000000000 ) ) ;
#893=CIRCLE ( 'NONE', #1742, 10.00000000000000178 ) ;
#896=DIRECTION ( 'NONE',  ( 0.000000000000000000, 0.000000000000000000, 1.000000000000000000 ) ) ;
#898=VERTEX_POINT ( 'NONE', #1955 ) ;
#899=EDGE_LOOP ( 'NONE', ( #1703, #7682 ) ) ;
#901=ORIENTED_EDGE ( 'NONE', *, *, #3298, .F. ) ;
#905=EDGE_CURVE ( 'NONE', #7935, #1253, #5191, .T. ) ;
#906=DIRECTION ( 'NONE',  ( 0.000000000000000000, -1.000000000000000000, 0.000000000000000000 ) ) ;
#908=ORIENTED_EDGE ( 'NONE', *, *, #1874, .F. ) ;
#909=CARTESIAN_POINT ( 'NONE',  ( -23.76520584195948516, -145.1457019118819005, 49.99999999999997868 ) ) ;
#913=ORIENTED_EDGE ( 'NONE', *, *, #10013, .T. ) ;
#916=DIRECTION ( 'NONE',  ( -0.7367503238654704578, 0.6761648913424330720, 0.000000000000000000 ) ) ;
#918=DIRECTION ( 'NONE',  ( -0.000000000000000000, -0.000000000000000000, -1.000000000000000000 ) ) ;
#919=CARTESIAN_POINT ( 'NONE',  ( 23.15769640663936002, -117.1457019118819005, -3.234176690190481738E-15 ) ) ;
#921=ADVANCED_FACE ( 'NONE', ( #8585 ), #1168, .T. ) ;
#924=DIRECTION ( 'NONE',  ( 1.000000000000000000, 0.000000000000000000, 0.000000000000000000 ) ) ;
#926=CYLINDRICAL_SURFACE ( 'NONE', #6588, 2.000000000000001776 ) ;
#927=ORIENTED_EDGE ( 'NONE', *, *, #103, .F. ) ;
#928=CIRCLE ( 'NONE', #6857, 2.000000000000001776 ) ;
#929=ORIENTED_EDGE ( 'NONE', *, *, #6063, .T. ) ;
#930=AXIS2_PLACEMENT_3D ( 'NONE', #9430, #3015, #2164 ) ;
#932=CARTESIAN_POINT ( 'NONE',  ( 39.99999999999997158, -135.1707019118818778, 43.99999999999997868 ) ) ;
#933=EDGE_CURVE ( 'NONE', #1886, #7639, #7594, .T. ) ;
#936=ADVANCED_FACE ( 'NONE', ( #9439 ), #3069, .F. ) ;
#939=VERTEX_POINT ( 'NONE', #4556 ) ;
#943=LINE ( 'NONE', #3385, #4422 ) ;
#944=AXIS2_PLACEMENT_3D ( 'NONE', #7492, #6536, #4207 ) ;
#947=CARTESIAN_POINT ( 'NONE',  ( 53.40242741783141156, 52.77167129626698028, 30.00000000000000355 ) ) ;
#948=VECTOR ( 'NONE', #9800, 1000.000000000000000 ) ;
#949=ADVANCED_FACE ( 'NONE', ( #5504 ), #7205, .T. ) ;
#951=ORIENTED_EDGE ( 'NONE', *, *, #10279, .F. ) ;
#953=AXIS2_PLACEMENT_3D ( 'NONE', #5208, #2131, #392 ) ;
#957=LINE ( 'NONE', #3504, #7581 ) ;
#963=AXIS2_PLACEMENT_3D ( 'NONE', #2254, #1408, #9464 ) ;
#964=EDGE_CURVE ( 'NONE', #1886, #6595, #6232, .T. ) ;
#965=AXIS2_PLACEMENT_3D ( 'NONE', #710, #3147, #6378 ) ;
#967=EDGE_LOOP ( 'NONE', ( #3889, #1251, #4780, #8395, #6209, #5356, #4672 ) ) ;
#968=FACE_OUTER_BOUND ( 'NONE', #5774, .T. ) ;
#969=CARTESIAN_POINT ( 'NONE',  ( 39.99999999999998579, -135.1457019118818721, -40.00000000000002132 ) ) ;
#971=CYLINDRICAL_SURFACE ( 'NONE', #9240, 2.000000000000001776 ) ;
#972=DIRECTION ( 'NONE',  ( 1.000000000000000000, 0.000000000000000000, -0.000000000000000000 ) ) ;
#974=LINE ( 'NONE', #1562, #1121 ) ;
#976=ORIENTED_EDGE ( 'NONE', *, *, #8479, .T. ) ;
#977=LINE ( 'NONE', #2569, #3578 ) ;
#979=VERTEX_POINT ( 'NONE', #8688 ) ;
#982=ORIENTED_EDGE ( 'NONE', *, *, #7902, .T. ) ;
#983=AXIS2_PLACEMENT_3D ( 'NONE', #6893, #2860, #6090 ) ;
#984=CARTESIAN_POINT ( 'NONE',  ( 0.000000000000000000, -115.1457019118818863, 49.99999999999997868 ) ) ;
#986=FACE_OUTER_BOUND ( 'NONE', #2888, .T. ) ;
#988=CARTESIAN_POINT ( 'NONE',  ( -27.15769640663939555, -133.1457019118818721, -27.15769640663944173 ) ) ;
#990=AXIS2_PLACEMENT_3D ( 'NONE', #4438, #1044, #2000 ) ;
#991=VERTEX_POINT ( 'NONE', #7996 ) ;
#994=EDGE_CURVE ( 'NONE', #9955, #2474, #3183, .T. ) ;
#995=EDGE_CURVE ( 'NONE', #8447, #1314, #3880, .T. ) ;
#996=VERTEX_POINT ( 'NONE', #688 ) ;
#997=CARTESIAN_POINT ( 'NONE',  ( 26.62179802177715615, -135.1457019118818721, -50.00000000000002132 ) ) ;
#999=CARTESIAN_POINT ( 'NONE',  ( -25.15769640663939199, -115.1457019118818863, -27.15769640663944173 ) ) ;
#1001=CARTESIAN_POINT ( 'NONE',  ( -40.00000000000002842, -135.1457019118818721, 49.99999999999997868 ) ) ;
#1002=DIRECTION ( 'NONE',  ( 0.000000000000000000, 1.000000000000000000, 0.000000000000000000 ) ) ;
#1005=VERTEX_POINT ( 'NONE', #3765 ) ;
#1007=EDGE_CURVE ( 'NONE', #1903, #826, #8841, .T. ) ;
#1009=EDGE_CURVE ( 'NONE', #59, #2261, #9804, .T. ) ;
#1010=AXIS2_PLACEMENT_3D ( 'NONE', #9428, #2213, #2270 ) ;
#1011=LINE ( 'NONE', #4973, #5882 ) ;
#1012=LINE ( 'NONE', #7373, #2929 ) ;
#1013=CARTESIAN_POINT ( 'NONE',  ( 25.15769640663936357, -115.1457019118818863, 27.15769640663938489 ) ) ;
#1014=ORIENTED_EDGE ( 'NONE', *, *, #5714, .T. ) ;
#1017=DIRECTION ( 'NONE',  ( 0.000000000000000000, 0.000000000000000000, -1.000000000000000000 ) ) ;
#1018=ORIENTED_EDGE ( 'NONE', *, *, #2964, .T. ) ;
#1019=EDGE_CURVE ( 'NONE', #7279, #2698, #8604, .T. ) ;
#1024=DIRECTION ( 'NONE',  ( 0.000000000000000000, 1.000000000000000000, 0.000000000000000000 ) ) ;
#1026=EDGE_CURVE ( 'NONE', #8639, #6250, #10468, .T. ) ;
#1029=FACE_OUTER_BOUND ( 'NONE', #6004, .T. ) ;
#1030=EDGE_LOOP ( 'NONE', ( #7266, #4767, #8673, #8457 ) ) ;
#1031=DIRECTION ( 'NONE',  ( 1.277197683604454965E-16, -1.000000000000000000, 0.000000000000000000 ) ) ;
#1032=EDGE_LOOP ( 'NONE', ( #8944, #461, #7397, #6704 ) ) ;
#1033=CARTESIAN_POINT ( 'NONE',  ( 97.72361618343356326, -145.1457019118818721, 30.00000000000000000 ) ) ;
#1035=CYLINDRICAL_SURFACE ( 'NONE', #1256, 4.000000000000000000 ) ;
#1037=DIRECTION ( 'NONE',  ( -0.000000000000000000, 1.000000000000000000, -0.000000000000000000 ) ) ;
#1038=CARTESIAN_POINT ( 'NONE',  ( -2.293506896408097795, 152.5696653505793279, -12.50000000000000000 ) ) ;
#1041=VECTOR ( 'NONE', #1434, 1000.000000000000000 ) ;
#1044=DIRECTION ( 'NONE',  ( 0.000000000000000000, -1.000000000000000000, 0.000000000000000000 ) ) ;
#1046=CARTESIAN_POINT ( 'NONE',  ( -23.15769640663940976, -135.1457019118818721, 49.99999999999997868 ) ) ;
#1048=CYLINDRICAL_SURFACE ( 'NONE', #1606, 31.75575292317714471 ) ;
#1051=VECTOR ( 'NONE', #4955, 1000.000000000000000 ) ;
#1055=ORIENTED_EDGE ( 'NONE', *, *, #5527, .F. ) ;
#1056=AXIS2_PLACEMENT_3D ( 'NONE', #10251, #6052, #6910 ) ;
#1058=AXIS2_PLACEMENT_3D ( 'NONE', #8553, #5110, #8811 ) ;
#1064=EDGE_CURVE ( 'NONE', #4776, #3587, #5889, .T. ) ;
#1065=LINE ( 'NONE', #5988, #7731 ) ;
#1073=VECTOR ( 'NONE', #55, 1000.000000000000114 ) ;
#1075=PLANE ( 'NONE',  #7656 ) ;
#1077=CYLINDRICAL_SURFACE ( 'NONE', #1290, 3.999999999999989786 ) ;
#1081=SHAPE_REPRESENTATION ( 'C-Frame Ductile Iron Housing', ( #4601 ), #9171 ) ;
#1086=ORIENTED_EDGE ( 'NONE', *, *, #8185, .T. ) ;
#1087=AXIS2_PLACEMENT_3D ( 'NONE', #9894, #296, #2715 ) ;
#1089=DIRECTION ( 'NONE',  ( -0.7367503238654704578, -0.6761648913424330720, 0.000000000000000000 ) ) ;
#1093=AXIS2_PLACEMENT_3D ( 'NONE', #10384, #8834, #7151 ) ;
#1094=LINE ( 'NONE', #313, #4102 ) ;
#1095=ORIENTED_EDGE ( 'NONE', *, *, #6186, .T. ) ;
#1097=CARTESIAN_POINT ( 'NONE',  ( -27.15769640663940976, -135.1457019118818721, 27.15769640663938489 ) ) ;
#1098=EDGE_CURVE ( 'NONE', #7848, #8983, #5864, .T. ) ;
#1104=DIRECTION ( 'NONE',  ( 0.000000000000000000, 0.000000000000000000, -1.000000000000000000 ) ) ;
#1106=CARTESIAN_POINT ( 'NONE',  ( 0.000000000000000000, -135.1457019118818721, -50.00000000000002132 ) ) ;
#1107=TOROIDAL_SURFACE ( 'NONE', #8212, 4.000000000000000000, 2.000000000000000000 ) ;
#1108=ORIENTED_EDGE ( 'NONE', *, *, #8919, .T. ) ;
#1113=CIRCLE ( 'NONE', #3829, 10.00000000000000178 ) ;
#1115=CARTESIAN_POINT ( 'NONE',  ( -40.00000000000001421, -145.1457019118819005, -36.00000000000002842 ) ) ;
#1121=VECTOR ( 'NONE', #863, 1000.000000000000000 ) ;
#1123=ORIENTED_EDGE ( 'NONE', *, *, #8274, .F. ) ;
#1127=AXIS2_PLACEMENT_3D ( 'NONE', #6102, #496, #5361 ) ;
#1130=DIRECTION ( 'NONE',  ( -0.000000000000000000, 1.000000000000000000, -0.000000000000000000 ) ) ;
#1133=DIRECTION ( 'NONE',  ( 0.000000000000000000, 0.000000000000000000, 1.000000000000000000 ) ) ;
#1136=TOROIDAL_SURFACE ( 'NONE', #6889, 26.75575292317714471, 5.000000000000000000 ) ;
#1137=EDGE_LOOP ( 'NONE', ( #3231, #9390, #5201, #9763 ) ) ;
#1139=ORIENTED_EDGE ( 'NONE', *, *, #1019, .F. ) ;
#1141=CIRCLE ( 'NONE', #800, 3.999999999999996447 ) ;
#1143=CARTESIAN_POINT ( 'NONE',  ( 37.50928405972917545, -135.0885866703937097, 26.66685298234238033 ) ) ;
#1145=DIRECTION ( 'NONE',  ( -1.000000000000000000, -0.000000000000000000, -0.000000000000000000 ) ) ;
#1149=VERTEX_POINT ( 'NONE', #4906 ) ;
#1155=ORIENTED_EDGE ( 'NONE', *, *, #7944, .F. ) ;
#1159=CARTESIAN_POINT ( 'NONE',  ( 23.15769640663939910, -117.1457019118819005, -48.00000000000002132 ) ) ;
#1162=DIRECTION ( 'NONE',  ( 0.000000000000000000, 0.000000000000000000, -1.000000000000000000 ) ) ;
#1168=CYLINDRICAL_SURFACE ( 'NONE', #6057, 2.000000000000001776 ) ;
#1169=DIRECTION ( 'NONE',  ( 1.277197683604454965E-16, -1.000000000000000000, 0.000000000000000000 ) ) ;
#1171=CARTESIAN_POINT ( 'NONE',  ( -50.00000000000001421, -135.1457019118818437, 26.27514435518735780 ) ) ;
#1172=DIRECTION ( 'NONE',  ( 8.659560562356134638E-17, 0.7071067811864494290, -0.7071067811866454944 ) ) ;
#1173=ORIENTED_EDGE ( 'NONE', *, *, #4710, .F. ) ;
#1174=CYLINDRICAL_SURFACE ( 'NONE', #6372, 2.000000000000001776 ) ;
#1177=EDGE_CURVE ( 'NONE', #9448, #1323, #8204, .T. ) ;
#1178=AXIS2_PLACEMENT_3D ( 'NONE', #4861, #5866, #5074 ) ;
#1179=ORIENTED_EDGE ( 'NONE', *, *, #1098, .T. ) ;
#1181=CARTESIAN_POINT ( 'NONE',  ( -2.293506896408101348, 37.08684478514406635, 25.00000000000000000 ) ) ;
#1185=CARTESIAN_POINT ( 'NONE',  ( 14.70649310359190309, 80.56966535057935630, -20.00000000000000711 ) ) ;
#1186=ORIENTED_EDGE ( 'NONE', *, *, #933, .F. ) ;
#1187=CARTESIAN_POINT ( 'NONE',  ( -23.76520584195948516, -145.1457019118819005, -50.00000000000002132 ) ) ;
#1188=EDGE_CURVE ( 'NONE', #2391, #1903, #4549, .T. ) ;
#1189=ORIENTED_EDGE ( 'NONE', *, *, #3064, .F. ) ;
#1191=ORIENTED_EDGE ( 'NONE', *, *, #6603, .T. ) ;
#1197=DIRECTION ( 'NONE',  ( 0.000000000000000000, -0.000000000000000000, 1.000000000000000000 ) ) ;
#1202=ORIENTED_EDGE ( 'NONE', *, *, #8903, .F. ) ;
#1204=CIRCLE ( 'NONE', #8813, 2.000000000000001776 ) ;
#1208=DIRECTION ( 'NONE',  ( 1.396588258780021135E-16, 0.000000000000000000, -1.000000000000000000 ) ) ;
#1209=DIRECTION ( 'NONE',  ( 0.000000000000000000, 0.000000000000000000, -1.000000000000000000 ) ) ;
#1211=LINE ( 'NONE', #1106, #9330 ) ;
#1212=AXIS2_PLACEMENT_3D ( 'NONE', #9106, #4907, #8097 ) ;
#1213=EDGE_CURVE ( 'NONE', #9582, #1239, #4026, .T. ) ;
#1214=ORIENTED_EDGE ( 'NONE', *, *, #10303, .F. ) ;
#1216=ORIENTED_EDGE ( 'NONE', *, *, #225, .F. ) ;
#1217=CARTESIAN_POINT ( 'NONE',  ( -23.15769640663937423, -133.1457019118818721, -50.00000000000002132 ) ) ;
#1218=VERTEX_POINT ( 'NONE', #997 ) ;
#1221=CYLINDRICAL_SURFACE ( 'NONE', #8153, 4.999999999999997335 ) ;
#1222=VECTOR ( 'NONE', #6537, 1000.000000000000114 ) ;
#1224=CARTESIAN_POINT ( 'NONE',  ( -16.29350689640809691, -186.9457019118818835, -27.01918567566963247 ) ) ;
#1226=ORIENTED_EDGE ( 'NONE', *, *, #994, .F. ) ;
#1227=ORIENTED_EDGE ( 'NONE', *, *, #7289, .T. ) ;
#1228=AXIS2_PLACEMENT_3D ( 'NONE', #1345, #6962, #2821 ) ;
#1231=EDGE_LOOP ( 'NONE', ( #908, #3006, #6193, #9020 ) ) ;
#1232=CARTESIAN_POINT ( 'NONE',  ( 17.97972049165455388, 37.08684478514406635, 30.00000000000000355 ) ) ;
#1239=VERTEX_POINT ( 'NONE', #160 ) ;
#1242=CARTESIAN_POINT ( 'NONE',  ( -40.00000000000001421, -135.1707019118818778, -40.00000000000002132 ) ) ;
#1245=DIRECTION ( 'NONE',  ( -1.000000000000000000, 0.000000000000000000, 0.000000000000000000 ) ) ;
#1248=DIRECTION ( 'NONE',  ( 0.000000000000000000, 0.000000000000000000, 1.000000000000000000 ) ) ;
#1250=CARTESIAN_POINT ( 'NONE',  ( -40.00000000000001421, -115.1457019118818863, -40.00000000000002132 ) ) ;
#1251=ORIENTED_EDGE ( 'NONE', *, *, #4194, .T. ) ;
#1253=VERTEX_POINT ( 'NONE', #6505 ) ;
#1254=DIRECTION ( 'NONE',  ( 0.000000000000000000, -0.000000000000000000, 1.000000000000000000 ) ) ;
#1255=ORIENTED_EDGE ( 'NONE', *, *, #475, .T. ) ;
#1256=AXIS2_PLACEMENT_3D ( 'NONE', #4271, #9252, #4325 ) ;
#1257=ORIENTED_EDGE ( 'NONE', *, *, #4817, .F. ) ;
#1260=DIRECTION ( 'NONE',  ( 1.000000000000000000, 0.000000000000000000, -0.000000000000000000 ) ) ;
#1261=ADVANCED_FACE ( 'NONE', ( #3434 ), #6878, .T. ) ;
#1262=EDGE_CURVE ( 'NONE', #4871, #8587, #6077, .T. ) ;
#1267=AXIS2_PLACEMENT_3D ( 'NONE', #9632, #508, #5320 ) ;
#1269=ORIENTED_EDGE ( 'NONE', *, *, #5144, .T. ) ;
#1271=AXIS2_PLACEMENT_3D ( 'NONE', #6457, #8000, #8045 ) ;
#1273=DIRECTION ( 'NONE',  ( 0.000000000000000000, 0.7071067811864494290, 0.7071067811866454944 ) ) ;
#1274=CARTESIAN_POINT ( 'NONE',  ( 42.22511195853866894, 17.84145331825995484, -25.00000000000000355 ) ) ;
#1275=EDGE_CURVE ( 'NONE', #6869, #10235, #6919, .T. ) ;
#1277=DIRECTION ( 'NONE',  ( 0.000000000000000000, 0.000000000000000000, -1.000000000000000000 ) ) ;
#1280=ORIENTED_EDGE ( 'NONE', *, *, #4742, .F. ) ;
#1285=DIRECTION ( 'NONE',  ( 0.000000000000000000, -0.000000000000000000, -1.000000000000000000 ) ) ;
#1286=CARTESIAN_POINT ( 'NONE',  ( 59.99999999999997868, -145.1457019118819005, 30.00000000000000355 ) ) ;
#1287=DIRECTION ( 'NONE',  ( 1.000000000000000000, 0.000000000000000000, -0.000000000000000000 ) ) ;
#1288=AXIS2_PLACEMENT_3D ( 'NONE', #6719, #5175, #10061 ) ;
#1290=AXIS2_PLACEMENT_3D ( 'NONE', #2028, #2769, #4415 ) ;
#1293=EDGE_CURVE ( 'NONE', #1886, #7279, #2790, .T. ) ;
#1294=CARTESIAN_POINT ( 'NONE',  ( -18.34874108452141783, -140.1746510883711778, -97.78965767959371647 ) ) ;
#1297=CARTESIAN_POINT ( 'NONE',  ( -50.00000000000002842, -135.1457019118818721, 39.99999999999997868 ) ) ;
#1298=CARTESIAN_POINT ( 'NONE',  ( 24.41868145091757825, -134.3099331815685105, -50.00000000000001421 ) ) ;
#1299=DIRECTION ( 'NONE',  ( 9.776117811460147207E-16, 0.000000000000000000, -1.000000000000000000 ) ) ;
#1301=ORIENTED_EDGE ( 'NONE', *, *, #3401, .T. ) ;
#1303=CIRCLE ( 'NONE', #9779, 2.000000000000001776 ) ;
#1304=VERTEX_POINT ( 'NONE', #2691 ) ;
#1306=EDGE_CURVE ( 'NONE', #7774, #6869, #7551, .T. ) ;
#1307=ORIENTED_EDGE ( 'NONE', *, *, #1584, .F. ) ;
#1308=LINE ( 'NONE', #6177, #5194 ) ;
#1310=CIRCLE ( 'NONE', #9272, 2.000000000000001776 ) ;
#1314=VERTEX_POINT ( 'NONE', #7515 ) ;
#1316=VECTOR ( 'NONE', #1172, 1000.000000000000000 ) ;
#1320=VECTOR ( 'NONE', #1750, 1000.000000000000000 ) ;
#1323=VERTEX_POINT ( 'NONE', #9105 ) ;
#1325=LINE ( 'NONE', #9490, #4345 ) ;
#1326=ORIENTED_EDGE ( 'NONE', *, *, #5527, .T. ) ;
#1329=ORIENTED_EDGE ( 'NONE', *, *, #3402, .T. ) ;
#1330=CARTESIAN_POINT ( 'NONE',  ( 37.59878849545336266, 37.08684478514405214, -12.50000000000000000 ) ) ;
#1332=LINE ( 'NONE', #9995, #7522 ) ;
#1335=ADVANCED_FACE ( 'NONE', ( #9320 ), #1892, .T. ) ;
#1338=ADVANCED_FACE ( 'NONE', ( #265 ), #10168, .F. ) ;
#1341=ORIENTED_EDGE ( 'NONE', *, *, #6759, .T. ) ;
#1342=DIRECTION ( 'NONE',  ( -1.000000000000000000, 0.000000000000000000, -0.000000000000000000 ) ) ;
#1343=FACE_OUTER_BOUND ( 'NONE', #311, .T. ) ;
#1345=CARTESIAN_POINT ( 'NONE',  ( 27.15769640663936713, -117.1457019118819005, 23.15769640663938134 ) ) ;
#1346=CARTESIAN_POINT ( 'NONE',  ( 0.000000000000000000, -135.1457019118818721, 0.000000000000000000 ) ) ;
#1348=VECTOR ( 'NONE', #6045, 1000.000000000000000 ) ;
#1349=CARTESIAN_POINT ( 'NONE',  ( 17.97972049165455388, 17.84145331825995484, 30.00000000000000355 ) ) ;
#1350=ADVANCED_FACE ( 'NONE', ( #2740 ), #3703, .T. ) ;
#1351=LINE ( 'NONE', #3687, #3374 ) ;
#1355=DIRECTION ( 'NONE',  ( -0.000000000000000000, -0.000000000000000000, -1.000000000000000000 ) ) ;
#1356=FACE_OUTER_BOUND ( 'NONE', #10389, .T. ) ;
#1358=DIRECTION ( 'NONE',  ( -0.000000000000000000, 1.000000000000000000, -0.000000000000000000 ) ) ;
#1361=ORIENTED_EDGE ( 'NONE', *, *, #5317, .F. ) ;
#1362=DIRECTION ( 'NONE',  ( 0.000000000000000000, 1.000000000000000000, 0.000000000000000000 ) ) ;
#1363=EDGE_LOOP ( 'NONE', ( #3684, #2571, #10349, #9047 ) ) ;
#1365=FACE_OUTER_BOUND ( 'NONE', #3229, .T. ) ;
#1366=SPHERICAL_SURFACE ( 'NONE', #6302, 2.000000000000000000 ) ;
#1374=DIRECTION ( 'NONE',  ( 0.000000000000000000, -1.000000000000000000, 0.000000000000000000 ) ) ;
#1376=ORIENTED_EDGE ( 'NONE', *, *, #3788, .T. ) ;
#1379=DIRECTION ( 'NONE',  ( -0.000000000000000000, 1.000000000000000000, 0.000000000000000000 ) ) ;
#1381=DIRECTION ( 'NONE',  ( 0.000000000000000000, 0.000000000000000000, 1.000000000000000000 ) ) ;
#1382=CIRCLE ( 'NONE', #2725, 2.000000000000001776 ) ;
#1385=ORIENTED_EDGE ( 'NONE', *, *, #287, .F. ) ;
#1387=AXIS2_PLACEMENT_3D ( 'NONE', #1488, #7206, #7899 ) ;
#1389=AXIS2_PLACEMENT_3D ( 'NONE', #3350, #4083, #9715 ) ;
#1392=DIRECTION ( 'NONE',  ( -0.000000000000000000, 1.000000000000000000, -0.000000000000000000 ) ) ;
#1394=CARTESIAN_POINT ( 'NONE',  ( 32.59878849545336976, 32.08684478514406635, 12.50000000000000355 ) ) ;
#1396=ADVANCED_FACE ( 'NONE', ( #3593 ), #9212, .F. ) ;
#1398=CARTESIAN_POINT ( 'NONE',  ( 14.70649310359190309, 80.56966535057935630, 16.00000000000000711 ) ) ;
#1401=TOROIDAL_SURFACE ( 'NONE', #8656, 4.000000000000000000, 2.000000000000000000 ) ;
#1408=DIRECTION ( 'NONE',  ( -0.7525569905852198538, -0.6585271261848804070, 0.000000000000000000 ) ) ;
#1409=DIRECTION ( 'NONE',  ( 0.000000000000000000, 0.000000000000000000, 1.000000000000000000 ) ) ;
#1410=CARTESIAN_POINT ( 'NONE',  ( 85.07264007511442117, 55.10093597859600578, 30.00000000000000355 ) ) ;
#1411=ORIENTED_EDGE ( 'NONE', *, *, #6341, .T. ) ;
#1412=CARTESIAN_POINT ( 'NONE',  ( 37.22511195853868315, -117.1457019118819005, 23.15769640663938134 ) ) ;
#1416=CARTESIAN_POINT ( 'NONE',  ( -16.29350689640809691, -140.1746510883711778, 27.01918567566963247 ) ) ;
#1417=ORIENTED_EDGE ( 'NONE', *, *, #8566, .F. ) ;
#1420=CARTESIAN_POINT ( 'NONE',  ( 10.51964330236497602, 150.0000000000000000, 12.50000000000000355 ) ) ;
#1422=DIRECTION ( 'NONE',  ( 1.000000000000000000, 0.000000000000000000, -0.000000000000000000 ) ) ;
#1423=DIRECTION ( 'NONE',  ( 0.000000000000000000, 0.000000000000000000, 1.000000000000000000 ) ) ;
#1425=DIRECTION ( 'NONE',  ( 0.000000000000000000, 1.000000000000000000, 0.000000000000000000 ) ) ;
#1429=VECTOR ( 'NONE', #8033, 1000.000000000000000 ) ;
#1431=PRODUCT_DEFINITION_FORMATION_WITH_SPECIFIED_SOURCE ( 'ANY', '', #2472, .NOT_KNOWN. ) ;
#1432=ORIENTED_EDGE ( 'NONE', *, *, #5788, .T. ) ;
#1433=DIRECTION ( 'NONE',  ( 0.000000000000000000, 0.000000000000000000, 1.000000000000000000 ) ) ;
#1434=DIRECTION ( 'NONE',  ( -0.000000000000000000, -0.000000000000000000, 1.000000000000000000 ) ) ;
#1437=CARTESIAN_POINT ( 'NONE',  ( 23.15769640663940265, -117.1457019118819005, -48.00000000000002132 ) ) ;
#1438=ORIENTED_EDGE ( 'NONE', *, *, #7942, .T. ) ;
#1446=VECTOR ( 'NONE', #164, 1000.000000000000000 ) ;
#1447=CARTESIAN_POINT ( 'NONE',  ( -20.14472382240651172, -141.8229441850657793, -28.16739522765907111 ) ) ;
#1449=DIRECTION ( 'NONE',  ( -1.000000000000000000, -0.000000000000000000, -0.000000000000000000 ) ) ;
#1451=DIRECTION ( 'NONE',  ( 0.000000000000000000, 0.000000000000000000, 1.000000000000000000 ) ) ;
#1456=EDGE_CURVE ( 'NONE', #9556, #5912, #2801, .T. ) ;
#1463=CARTESIAN_POINT ( 'NONE',  ( -40.00000000000001421, -135.1457019118818721, -44.00000000000001421 ) ) ;
#1465=DIRECTION ( 'NONE',  ( 0.000000000000000000, 0.000000000000000000, 1.000000000000000000 ) ) ;
#1469=VECTOR ( 'NONE', #602, 1000.000000000000000 ) ;
#1470=ADVANCED_FACE ( 'NONE', ( #1365 ), #4593, .T. ) ;
#1473=ORIENTED_EDGE ( 'NONE', *, *, #4035, .F. ) ;
#1474=DIRECTION ( 'NONE',  ( 0.000000000000000000, 0.000000000000000000, 1.000000000000000000 ) ) ;
#1475=CONICAL_SURFACE ( 'NONE', #10448, 4.025000000000000355, 0.7853981633975870569 ) ;
#1476=CYLINDRICAL_SURFACE ( 'NONE', #305, 2.000000000000001776 ) ;
#1478=DIRECTION ( 'NONE',  ( 1.000000000000000000, 0.000000000000000000, 8.379529552680125332E-16 ) ) ;
#1479=VECTOR ( 'NONE', #6419, 1000.000000000000000 ) ;
#1486=ORIENTED_EDGE ( 'NONE', *, *, #3167, .T. ) ;
#1487=DIRECTION ( 'NONE',  ( 0.000000000000000000, 1.000000000000000000, 0.000000000000000000 ) ) ;
#1488=CARTESIAN_POINT ( 'NONE',  ( 17.97972049165455388, 17.84145331825995484, 25.00000000000000000 ) ) ;
#1491=EDGE_CURVE ( 'NONE', #5933, #4432, #4268, .T. ) ;
#1493=AXIS2_PLACEMENT_3D ( 'NONE', #9562, #3939, #4675 ) ;
#1495=EDGE_LOOP ( 'NONE', ( #1173, #10130, #3801, #3859 ) ) ;
#1496=ORIENTED_EDGE ( 'NONE', *, *, #7467, .T. ) ;
#1497=AXIS2_PLACEMENT_3D ( 'NONE', #4715, #3173, #2224 ) ;
#1499=CARTESIAN_POINT ( 'NONE',  ( -50.00000000000002132, -134.6884840344297913, -24.98777100551304997 ) ) ;
#1500=DIRECTION ( 'NONE',  ( 0.000000000000000000, -1.000000000000000000, 0.000000000000000000 ) ) ;
#1502=CARTESIAN_POINT ( 'NONE',  ( 80.08610854271792334, 54.73418909528891874, -30.00000000000000355 ) ) ;
#1504=ORIENTED_EDGE ( 'NONE', *, *, #3206, .T. ) ;
#1505=CYLINDRICAL_SURFACE ( 'NONE', #3325, 10.00000000000000178 ) ;
#1506=AXIS2_PLACEMENT_3D ( 'NONE', #8795, #1487, #7898 ) ;
#1515=CARTESIAN_POINT ( 'NONE',  ( 24.98777100551300023, -134.6884840344297913, -50.00000000000002132 ) ) ;
#1518=VERTEX_POINT ( 'NONE', #9535 ) ;
#1521=ORIENTED_EDGE ( 'NONE', *, *, #4504, .F. ) ;
#1524=ORIENTED_EDGE ( 'NONE', *, *, #475, .F. ) ;
#1527=( NAMED_UNIT ( * ) SI_UNIT ( $, .STERADIAN. ) SOLID_ANGLE_UNIT ( ) );
#1530=EDGE_CURVE ( 'NONE', #9884, #109, #7194, .T. ) ;
#1533=CARTESIAN_POINT ( 'NONE',  ( 14.70649310359190309, 120.5696653505793705, 16.00000000000000711 ) ) ;
#1534=LINE ( 'NONE', #1625, #6676 ) ;
#1547=ORIENTED_EDGE ( 'NONE', *, *, #2111, .F. ) ;
#1548=CYLINDRICAL_SURFACE ( 'NONE', #5033, 4.999999999999997335 ) ;
#1549=CARTESIAN_POINT ( 'NONE',  ( -24.98775663295400662, -134.6884760388430777, -50.00000000000001421 ) ) ;
#1551=ORIENTED_EDGE ( 'NONE', *, *, #6866, .F. ) ;
#1553=CIRCLE ( 'NONE', #3938, 5.000000000000000888 ) ;
#1557=DIRECTION ( 'NONE',  ( 1.000000000000000000, 1.277197683604454965E-16, -0.000000000000000000 ) ) ;
#1559=VECTOR ( 'NONE', #1130, 1000.000000000000000 ) ;
#1561=DIRECTION ( 'NONE',  ( 0.000000000000000000, 0.000000000000000000, 1.000000000000000000 ) ) ;
#1562=CARTESIAN_POINT ( 'NONE',  ( 23.15769640663940265, -115.1457019118818863, -50.00000000000002132 ) ) ;
#1563=VERTEX_POINT ( 'NONE', #8284 ) ;
#1567=AXIS2_PLACEMENT_3D ( 'NONE', #5827, #222, #9063 ) ;
#1569=ADVANCED_FACE ( 'NONE', ( #185 ), #5941, .F. ) ;
#1572=CARTESIAN_POINT ( 'NONE',  ( -40.00000000000002842, -135.1707019118818778, 35.99999999999998579 ) ) ;
#1575=CARTESIAN_POINT ( 'NONE',  ( 2.108096605167895612E-14, -115.1457019118818863, -25.15769640663941686 ) ) ;
#1576=AXIS2_PLACEMENT_3D ( 'NONE', #2546, #119, #5722 ) ;
#1577=DIRECTION ( 'NONE',  ( -0.000000000000000000, 0.000000000000000000, -1.000000000000000000 ) ) ;
#1578=CYLINDRICAL_SURFACE ( 'NONE', #3499, 4.999999999999995559 ) ;
#1579=ORIENTED_EDGE ( 'NONE', *, *, #554, .F. ) ;
#1580=LINE ( 'NONE', #733, #9781 ) ;
#1581=EDGE_CURVE ( 'NONE', #7949, #5630, #3311, .T. ) ;
#1582=ADVANCED_FACE ( 'NONE', ( #9185 ), #971, .T. ) ;
#1584=EDGE_CURVE ( 'NONE', #8, #5946, #776, .T. ) ;
#1585=ORIENTED_EDGE ( 'NONE', *, *, #4551, .T. ) ;
#1589=CARTESIAN_POINT ( 'NONE',  ( -27.15769640663940976, -117.1457019118819005, 27.15769640663938489 ) ) ;
#1591=CIRCLE ( 'NONE', #416, 5.000000000000000888 ) ;
#1592=ORIENTED_EDGE ( 'NONE', *, *, #9396, .F. ) ;
#1595=CARTESIAN_POINT ( 'NONE',  ( -50.00000000000002132, -133.1457019118818721, -23.15769640663945594 ) ) ;
#1598=DIRECTION ( 'NONE',  ( -1.000000000000000000, -0.000000000000000000, -0.000000000000000000 ) ) ;
#1599=DIRECTION ( 'NONE',  ( 1.000000000000000000, 0.000000000000000000, 0.000000000000000000 ) ) ;
#1602=ORIENTED_EDGE ( 'NONE', *, *, #2681, .T. ) ;
#1604=AXIS2_PLACEMENT_3D ( 'NONE', #9056, #7466, #9761 ) ;
#1605=VERTEX_POINT ( 'NONE', #4307 ) ;
#1606=AXIS2_PLACEMENT_3D ( 'NONE', #947, #4286, #1743 ) ;
#1608=DIRECTION ( 'NONE',  ( 0.000000000000000000, 0.000000000000000000, -1.000000000000000000 ) ) ;
#1609=DIRECTION ( 'NONE',  ( -1.000000000000000000, 0.000000000000000000, 0.000000000000000000 ) ) ;
#1611=ADVANCED_FACE ( 'NONE', ( #3517 ), #6691, .F. ) ;
#1612=CARTESIAN_POINT ( 'NONE',  ( 37.29914372356918051, -134.6755117440382605, -25.86262238874442687 ) ) ;
#1614=CARTESIAN_POINT ( 'NONE',  ( 0.000000000000000000, -135.1457019118818721, 27.15769640663938489 ) ) ;
#1615=ORIENTED_EDGE ( 'NONE', *, *, #3498, .T. ) ;
#1622=CARTESIAN_POINT ( 'NONE',  ( -48.00000000000002132, -135.1457019118818721, 25.15769640663938134 ) ) ;
#1623=VECTOR ( 'NONE', #5440, 1000.000000000000000 ) ;
#1625=CARTESIAN_POINT ( 'NONE',  ( 25.15769640663937778, -117.1457019118819005, -25.15769640663940976 ) ) ;
#1628=VECTOR ( 'NONE', #1716, 1000.000000000000000 ) ;
#1631=VECTOR ( 'NONE', #6051, 1000.000000000000000 ) ;
#1634=DIRECTION ( 'NONE',  ( -0.000000000000000000, -0.000000000000000000, -1.000000000000000000 ) ) ;
#1636=CARTESIAN_POINT ( 'NONE',  ( 38.19229777560031636, 118.3760186273086816, 30.00000000000000355 ) ) ;
#1639=DIRECTION ( 'NONE',  ( 1.000000000000000000, 0.000000000000000000, 6.982941293900099513E-16 ) ) ;
#1642=VECTOR ( 'NONE', #6073, 1000.000000000000000 ) ;
#1643=EDGE_CURVE ( 'NONE', #4089, #6869, #3464, .T. ) ;
#1647=ORIENTED_EDGE ( 'NONE', *, *, #7, .F. ) ;
#1649=DIRECTION ( 'NONE',  ( -0.000000000000000000, 0.000000000000000000, 1.000000000000000000 ) ) ;
#1651=LINE ( 'NONE', #6320, #5962 ) ;
#1656=EDGE_CURVE ( 'NONE', #2182, #847, #9132, .T. ) ;
#1657=ADVANCED_FACE ( 'NONE', ( #2713 ), #8398, .T. ) ;
#1658=VERTEX_POINT ( 'NONE', #5152 ) ;
#1664=CARTESIAN_POINT ( 'NONE',  ( 0.000000000000000000, -135.1457019118818721, 30.00000000000000355 ) ) ;
#1670=VERTEX_POINT ( 'NONE', #9028 ) ;
#1673=CARTESIAN_POINT ( 'NONE',  ( -25.93999053166054480, -135.0799163051958942, 49.99999999999999289 ) ) ;
#1674=ORIENTED_EDGE ( 'NONE', *, *, #9568, .F. ) ;
#1679=CARTESIAN_POINT ( 'NONE',  ( 27.15769640663936713, -135.1457019118818721, 27.15769640663938489 ) ) ;
#1687=EDGE_CURVE ( 'NONE', #6849, #5630, #2077, .T. ) ;
#1690=CARTESIAN_POINT ( 'NONE',  ( 0.000000000000000000, -117.1457019118819005, 23.15769640663938134 ) ) ;
#1694=EDGE_LOOP ( 'NONE', ( #5212, #3936, #7368, #49 ) ) ;
#1696=EDGE_CURVE ( 'NONE', #6030, #4567, #3781, .T. ) ;
#1698=DIRECTION ( 'NONE',  ( 1.000000000000000000, 0.000000000000000000, 0.000000000000000000 ) ) ;
#1699=DIRECTION ( 'NONE',  ( 0.000000000000000000, 0.000000000000000000, 1.000000000000000000 ) ) ;
#1700=LINE ( 'NONE', #1013, #639 ) ;
#1701=ORIENTED_EDGE ( 'NONE', *, *, #10367, .F. ) ;
#1703=ORIENTED_EDGE ( 'NONE', *, *, #6039, .T. ) ;
#1705=EDGE_LOOP ( 'NONE', ( #2413, #6183, #5141, #2782, #6435, #883, #5365 ) ) ;
#1709=EDGE_CURVE ( 'NONE', #5357, #9948, #9345, .T. ) ;
#1713=DIRECTION ( 'NONE',  ( -1.000000000000000000, 0.000000000000000000, 1.396588258780020149E-16 ) ) ;
#1715=DIRECTION ( 'NONE',  ( 1.000000000000000000, 0.000000000000000000, 0.000000000000000000 ) ) ;
#1716=DIRECTION ( 'NONE',  ( 0.000000000000000000, 0.7071067811864494290, 0.7071067811866454944 ) ) ;
#1720=DIRECTION ( 'NONE',  ( -0.000000000000000000, 1.000000000000000000, -0.000000000000000000 ) ) ;
#1723=PLANE ( 'NONE',  #825 ) ;
#1724=ORIENTED_EDGE ( 'NONE', *, *, #8711, .T. ) ;
#1725=CIRCLE ( 'NONE', #10190, 2.000000000000001776 ) ;
#1726=ADVANCED_FACE ( 'NONE', ( #10036 ), #446, .F. ) ;
#1727=AXIS2_PLACEMENT_3D ( 'NONE', #6580, #1649, #1698 ) ;
#1730=DIRECTION ( 'NONE',  ( -1.000000000000000000, -0.000000000000000000, -0.000000000000000000 ) ) ;
#1735=ORIENTED_EDGE ( 'NONE', *, *, #5397, .F. ) ;
#1739=AXIS2_PLACEMENT_3D ( 'NONE', #2928, #9239, #10092 ) ;
#1740=LINE ( 'NONE', #1636, #7953 ) ;
#1741=CARTESIAN_POINT ( 'NONE',  ( -23.15769640663940976, -135.1457019118818721, 47.99999999999997868 ) ) ;
#1742=AXIS2_PLACEMENT_3D ( 'NONE', #4654, #5446, #6243 ) ;
#1743=DIRECTION ( 'NONE',  ( -1.000000000000000000, 0.000000000000000000, 0.000000000000000000 ) ) ;
#1747=EDGE_LOOP ( 'NONE', ( #1592, #5328, #555, #6139, #7007, #1929 ) ) ;
#1749=ORIENTED_EDGE ( 'NONE', *, *, #10145, .T. ) ;
#1750=DIRECTION ( 'NONE',  ( -1.387778780781445676E-16, 0.000000000000000000, 1.000000000000000000 ) ) ;
#1751=CARTESIAN_POINT ( 'NONE',  ( 37.22759939293836595, -117.1457019118819005, -25.15769640663939910 ) ) ;
#1752=DIRECTION ( 'NONE',  ( 1.000000000000000000, 0.000000000000000000, 0.000000000000000000 ) ) ;
#1753=CARTESIAN_POINT ( 'NONE',  ( -2.293506896408094242, 37.08684478514405214, 12.50000000000000000 ) ) ;
#1756=CARTESIAN_POINT ( 'NONE',  ( 37.22759939293836595, -117.1457019118819005, -25.15769640663939910 ) ) ;
#1759=ADVANCED_FACE ( 'NONE', ( #546 ), #9295, .F. ) ;
#1761=ORIENTED_EDGE ( 'NONE', *, *, #7993, .T. ) ;
#1763=DIRECTION ( 'NONE',  ( 0.000000000000000000, 0.000000000000000000, 1.000000000000000000 ) ) ;
#1766=DIRECTION ( 'NONE',  ( 0.000000000000000000, 0.000000000000000000, 1.000000000000000000 ) ) ;
#1774=EDGE_CURVE ( 'NONE', #5946, #8972, #6214, .T. ) ;
#1777=CARTESIAN_POINT ( 'NONE',  ( 27.15769640663940621, -133.1457019118818721, -48.00000000000002132 ) ) ;
#1778=ORIENTED_EDGE ( 'NONE', *, *, #3266, .T. ) ;
#1779=VECTOR ( 'NONE', #9160, 1000.000000000000000 ) ;
#1780=CARTESIAN_POINT ( 'NONE',  ( 27.15769640663938489, -133.1457019118818721, -27.15769640663940976 ) ) ;
#1782=DIRECTION ( 'NONE',  ( 0.000000000000000000, 0.000000000000000000, -1.000000000000000000 ) ) ;
#1783=DIRECTION ( 'NONE',  ( 0.000000000000000000, 0.000000000000000000, -1.000000000000000000 ) ) ;
#1787=EDGE_CURVE ( 'NONE', #2404, #9616, #2988, .T. ) ;
#1790=CARTESIAN_POINT ( 'NONE',  ( 25.15769640663936713, -133.1457019118818721, 47.99999999999997868 ) ) ;
#1794=AXIS2_PLACEMENT_3D ( 'NONE', #293, #4256, #3409 ) ;
#1795=CARTESIAN_POINT ( 'NONE',  ( -40.00000000000002842, -115.1457019118818863, 49.99999999999997868 ) ) ;
#1797=LINE ( 'NONE', #56, #10081 ) ;
#1799=EDGE_CURVE ( 'NONE', #2463, #4407, #3321, .T. ) ;
#1800=VERTEX_POINT ( 'NONE', #4571 ) ;
#1801=ORIENTED_EDGE ( 'NONE', *, *, #3926, .T. ) ;
#1802=VECTOR ( 'NONE', #5450, 1000.000000000000000 ) ;
#1806=ADVANCED_FACE ( 'NONE', ( #3623 ), #10091, .T. ) ;
#1807=CARTESIAN_POINT ( 'NONE',  ( 33.55285093437175448, 29.14909237014565946, 30.00000000000000355 ) ) ;
#1808=DIRECTION ( 'NONE',  ( 0.000000000000000000, 0.000000000000000000, 1.000000000000000000 ) ) ;
#1810=VECTOR ( 'NONE', #2046, 1000.000000000000000 ) ;
#1811=VERTEX_POINT ( 'NONE', #4822 ) ;
#1812=LINE ( 'NONE', #6786, #2141 ) ;
#1823=AXIS2_PLACEMENT_3D ( 'NONE', #234, #3460, #4885 ) ;
#1825=DIRECTION ( 'NONE',  ( -1.000000000000000000, 0.000000000000000000, 0.000000000000000000 ) ) ;
#1826=CONICAL_SURFACE ( 'NONE', #6683, 4.025000000000000355, 0.7853981633975870569 ) ;
#1827=ORIENTED_EDGE ( 'NONE', *, *, #4004, .T. ) ;
#1828=FACE_OUTER_BOUND ( 'NONE', #10076, .T. ) ;
#1829=ORIENTED_EDGE ( 'NONE', *, *, #9438, .T. ) ;
#1835=FACE_OUTER_BOUND ( 'NONE', #7369, .T. ) ;
#1843=EDGE_CURVE ( 'NONE', #8639, #4912, #3087, .T. ) ;
#1846=EDGE_CURVE ( 'NONE', #4360, #2186, #6492, .T. ) ;
#1847=LINE ( 'NONE', #1795, #5904 ) ;
#1848=CARTESIAN_POINT ( 'NONE',  ( -16.29350689640809691, -145.1457019118819005, 0.000000000000000000 ) ) ;
#1849=DIRECTION ( 'NONE',  ( 1.000000000000000000, 0.000000000000000000, -0.000000000000000000 ) ) ;
#1851=VECTOR ( 'NONE', #9375, 1000.000000000000000 ) ;
#1853=ORIENTED_EDGE ( 'NONE', *, *, #4817, .T. ) ;
#1855=CIRCLE ( 'NONE', #3209, 4.000000000000000000 ) ;
#1857=DIRECTION ( 'NONE',  ( 0.000000000000000000, 1.000000000000000000, 0.000000000000000000 ) ) ;
#1862=EDGE_LOOP ( 'NONE', ( #8414, #8544, #3619, #7668, #2073, #193 ) ) ;
#1868=CARTESIAN_POINT ( 'NONE',  ( 18.34874108452142494, -140.1746510883711778, -97.78965767959371647 ) ) ;
#1869=DIRECTION ( 'NONE',  ( -0.000000000000000000, 1.000000000000000000, -0.000000000000000000 ) ) ;
#1874=EDGE_CURVE ( 'NONE', #581, #2404, #7071, .T. ) ;
#1875=CARTESIAN_POINT ( 'NONE',  ( 18.34874108452142494, -140.1746510883711778, -50.00000000000002132 ) ) ;
#1879=FACE_OUTER_BOUND ( 'NONE', #967, .T. ) ;
#1882=CARTESIAN_POINT ( 'NONE',  ( 37.22511195853869026, -145.1457019118819005, 30.00000000000000355 ) ) ;
#1883=CIRCLE ( 'NONE', #5264, 5.000000000000000888 ) ;
#1884=CARTESIAN_POINT ( 'NONE',  ( 37.60382362833208703, -135.1346843322565121, 26.91340685820611611 ) ) ;
#1886=VERTEX_POINT ( 'NONE', #10456 ) ;
#1887=FACE_OUTER_BOUND ( 'NONE', #8797, .T. ) ;
#1892=CYLINDRICAL_SURFACE ( 'NONE', #8905, 2.000000000000001776 ) ;
#1893=CARTESIAN_POINT ( 'NONE',  ( 0.000000000000000000, -115.1457019118818863, 25.15769640663938134 ) ) ;
#1900=ORIENTED_EDGE ( 'NONE', *, *, #4631, .T. ) ;
#1901=ADVANCED_FACE ( 'NONE', ( #2389 ), #7124, .F. ) ;
#1903=VERTEX_POINT ( 'NONE', #1502 ) ;
#1904=EDGE_CURVE ( 'NONE', #1658, #5357, #701, .T. ) ;
#1905=CIRCLE ( 'NONE', #1739, 1.999999999999998224 ) ;
#1907=LINE ( 'NONE', #3556, #9287 ) ;
#1909=DIRECTION ( 'NONE',  ( 0.000000000000000000, 0.000000000000000000, 1.000000000000000000 ) ) ;
#1910=EDGE_LOOP ( 'NONE', ( #8695, #8822, #1055, #10301, #9500, #114, #7753, #6264 ) ) ;
#1912=VECTOR ( 'NONE', #8848, 1000.000000000000000 ) ;
#1914=CARTESIAN_POINT ( 'NONE',  ( -40.00000000000002842, -135.1707019118818778, 43.99999999999997868 ) ) ;
#1915=EDGE_CURVE ( 'NONE', #4722, #581, #3259, .T. ) ;
#1916=EDGE_LOOP ( 'NONE', ( #3525, #7798, #9101, #10095 ) ) ;
#1918=DIRECTION ( 'NONE',  ( 0.000000000000000000, 0.000000000000000000, -1.000000000000000000 ) ) ;
#1919=AXIS2_PLACEMENT_3D ( 'NONE', #2644, #9706, #211 ) ;
#1921=CARTESIAN_POINT ( 'NONE',  ( -23.76520584195948516, -145.1457019118819005, -50.00000000000002132 ) ) ;
#1923=DIRECTION ( 'NONE',  ( 1.000000000000000000, 0.000000000000000000, 0.000000000000000000 ) ) ;
#1927=ORIENTED_EDGE ( 'NONE', *, *, #2415, .F. ) ;
#1928=CARTESIAN_POINT ( 'NONE',  ( 0.000000000000000000, -133.1457019118818721, 27.15769640663938489 ) ) ;
#1929=ORIENTED_EDGE ( 'NONE', *, *, #1491, .F. ) ;
#1932=EDGE_CURVE ( 'NONE', #7949, #5111, #3020, .T. ) ;
#1933=AXIS2_PLACEMENT_3D ( 'NONE', #10415, #7768, #10210 ) ;
#1934=DIRECTION ( 'NONE',  ( 1.000000000000000000, 0.000000000000000000, 0.000000000000000000 ) ) ;
#1939=DIRECTION ( 'NONE',  ( 0.000000000000000000, 0.000000000000000000, 1.000000000000000000 ) ) ;
#1941=AXIS2_PLACEMENT_3D ( 'NONE', #3340, #7420, #8211 ) ;
#1943=ORIENTED_EDGE ( 'NONE', *, *, #9980, .T. ) ;
#1944=CARTESIAN_POINT ( 'NONE',  ( -27.15769640663940976, -133.1457019118818721, 27.15769640663938489 ) ) ;
#1947=CARTESIAN_POINT ( 'NONE',  ( 53.40242741783141156, 52.77167129626698028, -30.00000000000000355 ) ) ;
#1955=CARTESIAN_POINT ( 'NONE',  ( -2.293506896408097795, 147.5696653505793279, 30.00000000000000355 ) ) ;
#1958=FACE_OUTER_BOUND ( 'NONE', #8227, .T. ) ;
#1959=EDGE_CURVE ( 'NONE', #8659, #9556, #6246, .T. ) ;
#1961=EDGE_CURVE ( 'NONE', #9616, #3561, #1325, .T. ) ;
#1962=ORIENTED_EDGE ( 'NONE', *, *, #429, .T. ) ;
#1963=DIRECTION ( 'NONE',  ( 0.000000000000000000, 1.000000000000000000, 0.000000000000000000 ) ) ;
#1965=ORIENTED_EDGE ( 'NONE', *, *, #2549, .T. ) ;
#1967=VERTEX_POINT ( 'NONE', #478 ) ;
#1968=CARTESIAN_POINT ( 'NONE',  ( -25.15769640663940976, -117.1457019118819005, -1.756747170973246291E-14 ) ) ;
#1969=DIRECTION ( 'NONE',  ( 1.000000000000000000, 0.000000000000000000, 0.000000000000000000 ) ) ;
#1970=CIRCLE ( 'NONE', #4847, 7.500000000000000000 ) ;
#1979=EDGE_LOOP ( 'NONE', ( #4454, #3969, #492, #619 ) ) ;
#1982=ORIENTED_EDGE ( 'NONE', *, *, #1581, .F. ) ;
#1988=DIRECTION ( 'NONE',  ( 1.000000000000000000, 0.000000000000000000, 0.000000000000000000 ) ) ;
#1990=FACE_OUTER_BOUND ( 'NONE', #9713, .T. ) ;
#1991=CARTESIAN_POINT ( 'NONE',  ( 59.99999999999997868, -145.1457019118819005, 40.00000000000000000 ) ) ;
#1992=ORIENTED_EDGE ( 'NONE', *, *, #2654, .T. ) ;
#1995=ADVANCED_FACE ( 'NONE', ( #9275 ), #5398, .F. ) ;
#1996=ORIENTED_EDGE ( 'NONE', *, *, #5425, .T. ) ;
#1997=CIRCLE ( 'NONE', #6046, 3.297986701801175258 ) ;
#2000=DIRECTION ( 'NONE',  ( 0.000000000000000000, 0.000000000000000000, -1.000000000000000000 ) ) ;
#2003=DIRECTION ( 'NONE',  ( 1.000000000000000000, -0.000000000000000000, 0.000000000000000000 ) ) ;
#2005=AXIS2_PLACEMENT_3D ( 'NONE', #5768, #7427, #9118 ) ;
#2006=DIRECTION ( 'NONE',  ( 0.000000000000000000, 0.000000000000000000, 1.000000000000000000 ) ) ;
#2009=ORIENTED_EDGE ( 'NONE', *, *, #3968, .F. ) ;
#2010=CARTESIAN_POINT ( 'NONE',  ( -23.39899473324887680, -133.3869996355172987, -50.00000000000001421 ) ) ;
#2011=ORIENTED_EDGE ( 'NONE', *, *, #6309, .F. ) ;
#2012=CARTESIAN_POINT ( 'NONE',  ( 39.99999999999998579, -135.1457019118818721, -44.02500000000001990 ) ) ;
#2014=VECTOR ( 'NONE', #4092, 1000.000000000000000 ) ;
#2015=DIRECTION ( 'NONE',  ( 0.000000000000000000, -1.000000000000000000, 0.000000000000000000 ) ) ;
#2016=CARTESIAN_POINT ( 'NONE',  ( 17.97972049165455388, 37.08684478514406635, -12.49999999999997335 ) ) ;
#2017=VERTEX_POINT ( 'NONE', #6088 ) ;
#2020=CARTESIAN_POINT ( 'NONE',  ( -48.00000000000002132, -115.1457019118818863, -23.15769640663945594 ) ) ;
#2021=AXIS2_PLACEMENT_3D ( 'NONE', #6080, #8363, #4283 ) ;
#2024=DIRECTION ( 'NONE',  ( 0.000000000000000000, -1.000000000000000000, 0.000000000000000000 ) ) ;
#2025=CARTESIAN_POINT ( 'NONE',  ( -2.293506896408097795, 42.08684478514406635, -25.00000000000000355 ) ) ;
#2028=CARTESIAN_POINT ( 'NONE',  ( 39.99999999999997158, -135.1457019118818721, 39.99999999999997868 ) ) ;
#2029=ORIENTED_EDGE ( 'NONE', *, *, #5146, .F. ) ;
#2030=DIRECTION ( 'NONE',  ( 0.000000000000000000, 0.000000000000000000, -1.000000000000000000 ) ) ;
#2033=EDGE_CURVE ( 'NONE', #1605, #6079, #626, .T. ) ;
#2036=FACE_BOUND ( 'NONE', #4461, .T. ) ;
#2037=CARTESIAN_POINT ( 'NONE',  ( 37.23007123371004923, -133.6742494827832388, 25.22421275991299083 ) ) ;
#2042=DIRECTION ( 'NONE',  ( 1.000000000000000000, 0.000000000000000000, 0.000000000000000000 ) ) ;
#2044=ORIENTED_EDGE ( 'NONE', *, *, #10135, .T. ) ;
#2045=ADVANCED_FACE ( 'NONE', ( #2966 ), #6194, .T. ) ;
#2046=DIRECTION ( 'NONE',  ( 0.000000000000000000, -1.000000000000000000, 0.000000000000000000 ) ) ;
#2047=ORIENTED_EDGE ( 'NONE', *, *, #9769, .F. ) ;
#2048=AXIS2_PLACEMENT_3D ( 'NONE', #1868, #184, #916 ) ;
#2049=ORIENTED_EDGE ( 'NONE', *, *, #3138, .F. ) ;
#2050=CARTESIAN_POINT ( 'NONE',  ( 17.97972049165455388, 42.08684478514406635, -25.00000000000000000 ) ) ;
#2053=DIRECTION ( 'NONE',  ( -0.000000000000000000, 1.000000000000000000, -0.000000000000000000 ) ) ;
#2054=CARTESIAN_POINT ( 'NONE',  ( -2.293506896408097795, 152.5696653505793279, -24.99999999999998934 ) ) ;
#2068=ORIENTED_EDGE ( 'NONE', *, *, #3670, .F. ) ;
#2069=VERTEX_POINT ( 'NONE', #6450 ) ;
#2073=ORIENTED_EDGE ( 'NONE', *, *, #2722, .T. ) ;
#2074=ORIENTED_EDGE ( 'NONE', *, *, #5847, .F. ) ;
#2076=SPHERICAL_SURFACE ( 'NONE', #2568, 2.000000000000000000 ) ;
#2077=LINE ( 'NONE', #8491, #5687 ) ;
#2081=DIRECTION ( 'NONE',  ( 0.000000000000000000, -1.000000000000000000, 0.000000000000000000 ) ) ;
#2085=ORIENTED_EDGE ( 'NONE', *, *, #8968, .F. ) ;
#2087=PLANE ( 'NONE',  #9042 ) ;
#2088=EDGE_CURVE ( 'NONE', #10220, #2586, #9750, .T. ) ;
#2089=PLANE ( 'NONE',  #6695 ) ;
#2091=EDGE_CURVE ( 'NONE', #4437, #10082, #8793, .T. ) ;
#2092=ORIENTED_EDGE ( 'NONE', *, *, #8505, .T. ) ;
#2093=DIRECTION ( 'NONE',  ( -1.000000000000000000, -0.000000000000000000, -0.000000000000000000 ) ) ;
#2098=CARTESIAN_POINT ( 'NONE',  ( 77.30044127146538813, 73.68369600860394542, 25.00000000000000000 ) ) ;
#2100=ORIENTED_EDGE ( 'NONE', *, *, #3024, .F. ) ;
#2104=DIRECTION ( 'NONE',  ( -1.000000000000000000, 0.000000000000000000, -0.000000000000000000 ) ) ;
#2105=ORIENTED_EDGE ( 'NONE', *, *, #8613, .T. ) ;
#2106=CARTESIAN_POINT ( 'NONE',  ( -16.29350689640809691, -140.1746510883711778, -7.500000000000000000 ) ) ;
#2111=EDGE_CURVE ( 'NONE', #6094, #1253, #8920, .T. ) ;
#2113=TOROIDAL_SURFACE ( 'NONE', #6350, 4.000000000000000000, 2.000000000000000000 ) ;
#2115=DIRECTION ( 'NONE',  ( -1.000000000000000000, 0.000000000000000000, 0.000000000000000000 ) ) ;
#2119=DIRECTION ( 'NONE',  ( 0.000000000000000000, 0.000000000000000000, -1.000000000000000000 ) ) ;
#2120=CARTESIAN_POINT ( 'NONE',  ( 27.15769640663936713, -115.1457019118818863, 23.15769640663938134 ) ) ;
#2122=ORIENTED_EDGE ( 'NONE', *, *, #10086, .F. ) ;
#2123=ORIENTED_EDGE ( 'NONE', *, *, #5788, .F. ) ;
#2128=ORIENTED_EDGE ( 'NONE', *, *, #7497, .T. ) ;
#2129=CARTESIAN_POINT ( 'NONE',  ( -16.29350689640809691, -115.1457019118818863, 27.01918567566963247 ) ) ;
#2131=DIRECTION ( 'NONE',  ( -0.6585271261848815172, 0.7525569905852190766, -4.569449861441823711E-16 ) ) ;
#2132=LINE ( 'NONE', #8492, #9187 ) ;
#2134=CARTESIAN_POINT ( 'NONE',  ( -40.00000000000002842, -145.1457019118819005, 49.99999999999997868 ) ) ;
#2136=VERTEX_POINT ( 'NONE', #10338 ) ;
#2137=LINE ( 'NONE', #6271, #5610 ) ;
#2138=AXIS2_PLACEMENT_3D ( 'NONE', #427, #6890, #5241 ) ;
#2139=DIRECTION ( 'NONE',  ( 1.000000000000000000, 0.000000000000000000, 8.379529552680124346E-16 ) ) ;
#2141=VECTOR ( 'NONE', #10230, 1000.000000000000000 ) ;
#2142=DIRECTION ( 'NONE',  ( 0.000000000000000000, 0.000000000000000000, -1.000000000000000000 ) ) ;
#2144=CARTESIAN_POINT ( 'NONE',  ( -50.00000000000002132, -115.1457019118818863, -6.938893903907231533E-15 ) ) ;
#2147=DIRECTION ( 'NONE',  ( 1.396588258780021135E-16, 0.000000000000000000, 1.000000000000000000 ) ) ;
#2148=VECTOR ( 'NONE', #4795, 1000.000000000000000 ) ;
#2154=VERTEX_POINT ( 'NONE', #8739 ) ;
#2155=AXIS2_PLACEMENT_3D ( 'NONE', #7971, #21, #3044 ) ;
#2160=CARTESIAN_POINT ( 'NONE',  ( 14.70649310359190309, 80.56966535057935630, -20.00000000000000711 ) ) ;
#2161=EDGE_CURVE ( 'NONE', #3561, #6261, #3170, .T. ) ;
#2162=AXIS2_PLACEMENT_3D ( 'NONE', #9579, #10209, #2142 ) ;
#2164=DIRECTION ( 'NONE',  ( 0.000000000000000000, 0.000000000000000000, -1.000000000000000000 ) ) ;
#2165=DIRECTION ( 'NONE',  ( -0.000000000000000000, 1.000000000000000000, 0.000000000000000000 ) ) ;
#2166=DIRECTION ( 'NONE',  ( 1.000000000000000000, -0.000000000000000000, -0.000000000000000000 ) ) ;
#2169=CARTESIAN_POINT ( 'NONE',  ( 23.15769640663940265, -115.1457019118818863, -48.00000000000002132 ) ) ;
#2170=EDGE_CURVE ( 'NONE', #5671, #2596, #7914, .T. ) ;
#2171=EDGE_CURVE ( 'NONE', #8901, #3840, #9435, .T. ) ;
#2174=DIRECTION ( 'NONE',  ( 0.000000000000000000, 0.000000000000000000, 1.000000000000000000 ) ) ;
#2175=CARTESIAN_POINT ( 'NONE',  ( 27.15769640663936713, -117.1457019118819005, 27.15769640663938489 ) ) ;
#2177=SPHERICAL_SURFACE ( 'NONE', #3783, 2.000000000000000000 ) ;
#2178=CARTESIAN_POINT ( 'NONE',  ( -2.293506896408097795, 152.5696653505793279, -30.00000000000000355 ) ) ;
#2179=CARTESIAN_POINT ( 'NONE',  ( 38.19229777560031636, -43.28483205141633761, -12.50000000000000000 ) ) ;
#2181=ORIENTED_EDGE ( 'NONE', *, *, #3367, .F. ) ;
#2182=VERTEX_POINT ( 'NONE', #4752 ) ;
#2184=EDGE_CURVE ( 'NONE', #7051, #7422, #1580, .T. ) ;
#2185=VECTOR ( 'NONE', #4044, 1000.000000000000000 ) ;
#2186=VERTEX_POINT ( 'NONE', #4804 ) ;
#2187=CARTESIAN_POINT ( 'NONE',  ( -2.293506896408097795, 152.5696653505793279, 30.00000000000000355 ) ) ;
#2191=LINE ( 'NONE', #3038, #1469 ) ;
#2193=CIRCLE ( 'NONE', #3040, 4.000000000000000000 ) ;
#2196=ORIENTED_EDGE ( 'NONE', *, *, #7267, .T. ) ;
#2197=LINE ( 'NONE', #2831, #9091 ) ;
#2199=DIRECTION ( 'NONE',  ( 0.000000000000000000, 0.000000000000000000, -1.000000000000000000 ) ) ;
#2200=EDGE_CURVE ( 'NONE', #8048, #6849, #4023, .T. ) ;
#2203=CARTESIAN_POINT ( 'NONE',  ( 17.97972049165455388, 42.08684478514406635, 30.00000000000000355 ) ) ;
#2204=ORIENTED_EDGE ( 'NONE', *, *, #6543, .F. ) ;
#2208=ORIENTED_EDGE ( 'NONE', *, *, #4655, .F. ) ;
#2213=DIRECTION ( 'NONE',  ( -0.6761648913424331830, 0.7367503238654705688, 0.000000000000000000 ) ) ;
#2216=CARTESIAN_POINT ( 'NONE',  ( -25.15769640663937423, -117.1457019118819005, -48.00000000000002132 ) ) ;
#2217=CARTESIAN_POINT ( 'NONE',  ( 53.40242741783141156, 52.77167129626698028, 30.00000000000000355 ) ) ;
#2222=AXIS2_PLACEMENT_3D ( 'NONE', #6885, #2165, #9218 ) ;
#2224=DIRECTION ( 'NONE',  ( 0.000000000000000000, 0.000000000000000000, -1.000000000000000000 ) ) ;
#2225=FACE_BOUND ( 'NONE', #4473, .T. ) ;
#2226=ORIENTED_EDGE ( 'NONE', *, *, #1098, .F. ) ;
#2228=DIRECTION ( 'NONE',  ( 0.000000000000000000, 0.000000000000000000, 1.000000000000000000 ) ) ;
#2232=ORIENTED_EDGE ( 'NONE', *, *, #6583, .T. ) ;
#2236=EDGE_LOOP ( 'NONE', ( #1376, #7614, #1473, #10387 ) ) ;
#2240=CARTESIAN_POINT ( 'NONE',  ( -16.29350689640809691, -186.9457019118818835, 27.01918567566963247 ) ) ;
#2241=LINE ( 'NONE', #8648, #9006 ) ;
#2249=VECTOR ( 'NONE', #2042, 1000.000000000000000 ) ;
#2251=ORIENTED_EDGE ( 'NONE', *, *, #3281, .T. ) ;
#2254=CARTESIAN_POINT ( 'NONE',  ( 77.30044127146538813, 73.68369600860394542, 30.00000000000000355 ) ) ;
#2261=VERTEX_POINT ( 'NONE', #1790 ) ;
#2264=EDGE_CURVE ( 'NONE', #6316, #7078, #98, .T. ) ;
#2266=EDGE_LOOP ( 'NONE', ( #5185, #8963, #9468, #1255 ) ) ;
#2268=LINE ( 'NONE', #9479, #5275 ) ;
#2270=DIRECTION ( 'NONE',  ( -0.7367503238654704578, -0.6761648913424330720, 0.000000000000000000 ) ) ;
#2272=CARTESIAN_POINT ( 'NONE',  ( 23.15769640663936713, -135.1457019118818721, 47.99999999999997868 ) ) ;
#2273=CARTESIAN_POINT ( 'NONE',  ( 23.15769640663936713, -117.1457019118819005, 47.99999999999997868 ) ) ;
#2276=AXIS2_PLACEMENT_3D ( 'NONE', #5443, #4747, #3162 ) ;
#2280=EDGE_CURVE ( 'NONE', #47, #2630, #5172, .T. ) ;
#2281=DIRECTION ( 'NONE',  ( -0.000000000000000000, 1.000000000000000000, 0.000000000000000000 ) ) ;
#2282=LINE ( 'NONE', #5402, #1041 ) ;
#2284=FACE_OUTER_BOUND ( 'NONE', #1032, .T. ) ;
#2285=AXIS2_PLACEMENT_3D ( 'NONE', #5480, #1409, #7817 ) ;
#2286=LINE ( 'NONE', #5661, #8210 ) ;
#2294=CARTESIAN_POINT ( 'NONE',  ( 23.64290342185648797, -133.6308916829187297, 49.99999999999999289 ) ) ;
#2295=DIRECTION ( 'NONE',  ( 6.982941293900105430E-16, 0.000000000000000000, -1.000000000000000000 ) ) ;
#2297=DIRECTION ( 'NONE',  ( -0.000000000000000000, 0.000000000000000000, 1.000000000000000000 ) ) ;
#2298=ORIENTED_EDGE ( 'NONE', *, *, #5367, .T. ) ;
#2301=ORIENTED_EDGE ( 'NONE', *, *, #3837, .F. ) ;
#2303=CYLINDRICAL_SURFACE ( 'NONE', #965, 2.000000000000001776 ) ;
#2304=EDGE_CURVE ( 'NONE', #9783, #4360, #4173, .T. ) ;
#2305=AXIS2_PLACEMENT_3D ( 'NONE', #2560, #8387, #4365 ) ;
#2310=DIRECTION ( 'NONE',  ( -0.7525569905852205199, -0.6585271261848794078, 0.000000000000000000 ) ) ;
#2311=CARTESIAN_POINT ( 'NONE',  ( 42.22511195853866184, 52.77167129626698028, 25.00000000000000000 ) ) ;
#2313=LINE ( 'NONE', #2203, #4609 ) ;
#2314=VECTOR ( 'NONE', #7963, 1000.000000000000000 ) ;
#2318=DIRECTION ( 'NONE',  ( -1.000000000000000000, 0.000000000000000000, 0.000000000000000000 ) ) ;
#2319=ORIENTED_EDGE ( 'NONE', *, *, #905, .F. ) ;
#2322=VECTOR ( 'NONE', #5327, 1000.000000000000000 ) ;
#2323=DIRECTION ( 'NONE',  ( 0.000000000000000000, 0.000000000000000000, 1.000000000000000000 ) ) ;
#2324=CARTESIAN_POINT ( 'NONE',  ( 27.15769640663936713, -117.1457019118819005, 25.15769640663938134 ) ) ;
#2326=DIRECTION ( 'NONE',  ( 0.000000000000000000, 1.000000000000000000, -0.000000000000000000 ) ) ;
#2328=CARTESIAN_POINT ( 'NONE',  ( -50.00000000000001421, -135.1457019118818721, -40.00000000000002132 ) ) ;
#2330=DIRECTION ( 'NONE',  ( 1.000000000000000000, 0.000000000000000000, 0.000000000000000000 ) ) ;
#2333=DIRECTION ( 'NONE',  ( 1.000000000000000000, 0.000000000000000000, 1.387778780781445676E-16 ) ) ;
#2335=DIRECTION ( 'NONE',  ( 1.000000000000000000, 0.000000000000000000, 0.000000000000000000 ) ) ;
#2337=VECTOR ( 'NONE', #10307, 1000.000000000000000 ) ;
#2339=VERTEX_POINT ( 'NONE', #1097 ) ;
#2341=ORIENTED_EDGE ( 'NONE', *, *, #5916, .T. ) ;
#2344=CARTESIAN_POINT ( 'NONE',  ( 27.15769640663936713, -133.1457019118818721, 25.15769640663938134 ) ) ;
#2349=ORIENTED_EDGE ( 'NONE', *, *, #2669, .T. ) ;
#2351=ADVANCED_FACE ( 'NONE', ( #3543 ), #1136, .T. ) ;
#2355=CARTESIAN_POINT ( 'NONE',  ( 27.15769640663936713, -115.1457019118818863, 27.15769640663938489 ) ) ;
#2357=VERTEX_POINT ( 'NONE', #4279 ) ;
#2358=DIRECTION ( 'NONE',  ( 0.000000000000000000, 0.000000000000000000, 1.000000000000000000 ) ) ;
#2359=ADVANCED_FACE ( 'NONE', ( #8619 ), #1475, .F. ) ;
#2361=ADVANCED_FACE ( 'NONE', ( #9368 ), #10165, .T. ) ;
#2363=DIRECTION ( 'NONE',  ( 0.000000000000000000, 0.000000000000000000, -1.000000000000000000 ) ) ;
#2364=CIRCLE ( 'NONE', #8286, 4.000000000000000000 ) ;
#2366=CARTESIAN_POINT ( 'NONE',  ( -50.00000000000001421, -135.1457019118818721, -26.62179802177720944 ) ) ;
#2369=DIRECTION ( 'NONE',  ( -0.000000000000000000, -0.000000000000000000, -1.000000000000000000 ) ) ;
#2370=CARTESIAN_POINT ( 'NONE',  ( 80.08610854271792334, 54.73418909528891874, 25.00000000000000000 ) ) ;
#2371=EDGE_CURVE ( 'NONE', #1314, #3326, #1970, .T. ) ;
#2384=DIRECTION ( 'NONE',  ( -0.000000000000000000, 1.000000000000000000, -0.000000000000000000 ) ) ;
#2386=CARTESIAN_POINT ( 'NONE',  ( 24.98775663295400307, -134.6884760388430777, 49.99999999999998579 ) ) ;
#2387=ORIENTED_EDGE ( 'NONE', *, *, #6169, .F. ) ;
#2389=FACE_OUTER_BOUND ( 'NONE', #6953, .T. ) ;
#2391=VERTEX_POINT ( 'NONE', #2893 ) ;
#2393=EDGE_LOOP ( 'NONE', ( #10409, #10009, #5914, #216 ) ) ;
#2396=CONICAL_SURFACE ( 'NONE', #713, 4.025000000000000355, 0.7853981633975870569 ) ;
#2400=CIRCLE ( 'NONE', #10198, 3.999999999999989786 ) ;
#2401=AXIS2_PLACEMENT_3D ( 'NONE', #669, #1358, #1465 ) ;
#2402=DIRECTION ( 'NONE',  ( 0.000000000000000000, 0.000000000000000000, 1.000000000000000000 ) ) ;
#2403=CARTESIAN_POINT ( 'NONE',  ( 37.31847924783638604, -134.7590046800779930, -25.96838025129187599 ) ) ;
#2404=VERTEX_POINT ( 'NONE', #465 ) ;
#2405=CARTESIAN_POINT ( 'NONE',  ( -16.29350689640809691, -186.9457019118818835, 30.31717237747080773 ) ) ;
#2410=VECTOR ( 'NONE', #4214, 1000.000000000000000 ) ;
#2411=AXIS2_PLACEMENT_3D ( 'NONE', #2217, #3216, #9650 ) ;
#2413=ORIENTED_EDGE ( 'NONE', *, *, #7111, .F. ) ;
#2415=EDGE_CURVE ( 'NONE', #2815, #4536, #6126, .T. ) ;
#2417=DIRECTION ( 'NONE',  ( 0.000000000000000000, 0.000000000000000000, 1.000000000000000000 ) ) ;
#2418=CARTESIAN_POINT ( 'NONE',  ( 0.000000000000000000, -117.1457019118819005, 49.99999999999997868 ) ) ;
#2422=ORIENTED_EDGE ( 'NONE', *, *, #8582, .T. ) ;
#2424=VECTOR ( 'NONE', #2003, 1000.000000000000000 ) ;
#2427=EDGE_CURVE ( 'NONE', #2261, #7537, #514, .T. ) ;
#2429=EDGE_CURVE ( 'NONE', #6600, #2463, #1308, .T. ) ;
#2431=CARTESIAN_POINT ( 'NONE',  ( 39.99999999999997158, -145.1457019118819005, 49.99999999999997868 ) ) ;
#2434=CARTESIAN_POINT ( 'NONE',  ( -16.29350689640809691, -115.1457019118818863, -27.01918567566963247 ) ) ;
#2436=AXIS2_PLACEMENT_3D ( 'NONE', #10103, #1245, #7612 ) ;
#2443=EDGE_CURVE ( 'NONE', #2136, #6531, #8463, .T. ) ;
#2448=DIRECTION ( 'NONE',  ( 0.000000000000000000, -1.000000000000000000, 0.000000000000000000 ) ) ;
#2450=AXIS2_PLACEMENT_3D ( 'NONE', #1437, #4811, #791 ) ;
#2452=AXIS2_PLACEMENT_3D ( 'NONE', #7846, #10392, #3026 ) ;
#2455=CYLINDRICAL_SURFACE ( 'NONE', #3976, 2.000000000000001776 ) ;
#2456=CARTESIAN_POINT ( 'NONE',  ( 37.46807877396356190, -135.0538248752150139, -26.54476371764646103 ) ) ;
#2462=CARTESIAN_POINT ( 'NONE',  ( -38.19229777560033057, 152.5696653505793279, -12.50000000000000000 ) ) ;
#2463=VERTEX_POINT ( 'NONE', #6818 ) ;
#2465=ORIENTED_EDGE ( 'NONE', *, *, #3079, .F. ) ;
#2470=CARTESIAN_POINT ( 'NONE',  ( -18.34874108452141783, -140.1746510883711778, -50.00000000000002132 ) ) ;
#2471=DIRECTION ( 'NONE',  ( -1.000000000000000000, -1.734723475976805319E-15, -0.000000000000000000 ) ) ;
#2472=PRODUCT ( 'C-Frame Ductile Iron Housing', 'C-Frame Ductile Iron Housing', '', ( #192 ) ) ;
#2474=VERTEX_POINT ( 'NONE', #413 ) ;
#2476=EDGE_LOOP ( 'NONE', ( #704, #3245, #648, #8165, #2567, #2846, #1417, #1179, #5247, #9908, #8106, #2341 ) ) ;
#2477=CARTESIAN_POINT ( 'NONE',  ( 14.70649310359190309, 120.5696653505793705, 16.00000000000000711 ) ) ;
#2478=FACE_OUTER_BOUND ( 'NONE', #3614, .T. ) ;
#2481=DIRECTION ( 'NONE',  ( 0.000000000000000000, 0.000000000000000000, 1.000000000000000000 ) ) ;
#2486=EDGE_CURVE ( 'NONE', #7639, #9939, #3645, .T. ) ;
#2489=EDGE_CURVE ( 'NONE', #2732, #5224, #4039, .T. ) ;
#2491=ORIENTED_EDGE ( 'NONE', *, *, #1774, .T. ) ;
#2497=AXIS2_PLACEMENT_3D ( 'NONE', #5723, #9930, #2548 ) ;
#2501=DIRECTION ( 'NONE',  ( 0.000000000000000000, 0.000000000000000000, -1.000000000000000000 ) ) ;
#2507=DIRECTION ( 'NONE',  ( 1.277197683604454965E-16, -1.000000000000000000, 0.000000000000000000 ) ) ;
#2508=FACE_BOUND ( 'NONE', #5851, .T. ) ;
#2510=DIRECTION ( 'NONE',  ( 0.000000000000000000, 0.000000000000000000, 1.000000000000000000 ) ) ;
#2511=VECTOR ( 'NONE', #9492, 1000.000000000000227 ) ;
#2514=VERTEX_POINT ( 'NONE', #8028 ) ;
#2517=ORIENTED_EDGE ( 'NONE', *, *, #3629, .F. ) ;
#2518=CARTESIAN_POINT ( 'NONE',  ( -27.15769640663941331, -135.1457019118818721, 47.99999999999997868 ) ) ;
#2523=DIRECTION ( 'NONE',  ( -1.000000000000000000, 0.000000000000000000, 0.000000000000000000 ) ) ;
#2524=CARTESIAN_POINT ( 'NONE',  ( 14.70649310359190309, 120.5696653505793705, 24.00000000000000711 ) ) ;
#2525=DIRECTION ( 'NONE',  ( 0.000000000000000000, -1.000000000000000000, 0.000000000000000000 ) ) ;
#2527=VECTOR ( 'NONE', #1208, 1000.000000000000000 ) ;
#2528=EDGE_LOOP ( 'NONE', ( #771, #5503, #4451, #7777, #2730, #8563 ) ) ;
#2537=CARTESIAN_POINT ( 'NONE',  ( 18.34874108452142494, -140.1746510883711778, 49.99999999999997868 ) ) ;
#2538=EDGE_LOOP ( 'NONE', ( #273, #1647, #3485, #1189 ) ) ;
#2542=VERTEX_POINT ( 'NONE', #7190 ) ;
#2544=DIRECTION ( 'NONE',  ( -0.000000000000000000, -0.000000000000000000, -1.000000000000000000 ) ) ;
#2546=CARTESIAN_POINT ( 'NONE',  ( 39.99999999999997158, -135.1457019118818721, 39.99999999999997868 ) ) ;
#2548=DIRECTION ( 'NONE',  ( 0.000000000000000000, 0.000000000000000000, -1.000000000000000000 ) ) ;
#2549=EDGE_CURVE ( 'NONE', #4432, #3359, #721, .T. ) ;
#2552=CYLINDRICAL_SURFACE ( 'NONE', #4180, 3.999999999999989786 ) ;
#2556=CIRCLE ( 'NONE', #6440, 1.999999999999998224 ) ;
#2560=CARTESIAN_POINT ( 'NONE',  ( 17.97972049165455388, 17.84145331825995484, -25.00000000000000355 ) ) ;
#2561=DIRECTION ( 'NONE',  ( -1.396588258780021135E-16, 0.000000000000000000, -1.000000000000000000 ) ) ;
#2562=EDGE_CURVE ( 'NONE', #9948, #9616, #9283, .T. ) ;
#2564=CARTESIAN_POINT ( 'NONE',  ( -27.15769640663941331, -133.1457019118818721, -1.896405996851248439E-14 ) ) ;
#2565=CARTESIAN_POINT ( 'NONE',  ( -40.00000000000001421, -135.1457019118818721, -40.00000000000002132 ) ) ;
#2566=AXIS2_PLACEMENT_3D ( 'NONE', #9000, #786, #5706 ) ;
#2567=ORIENTED_EDGE ( 'NONE', *, *, #5846, .T. ) ;
#2568=AXIS2_PLACEMENT_3D ( 'NONE', #5305, #10248, #6908 ) ;
#2569=CARTESIAN_POINT ( 'NONE',  ( 23.15769640663936002, -115.1457019118818863, -3.234176690190481738E-15 ) ) ;
#2571=ORIENTED_EDGE ( 'NONE', *, *, #9829, .T. ) ;
#2572=CARTESIAN_POINT ( 'NONE',  ( -26.27514770175547199, -135.1457019118818721, 49.99999999999998579 ) ) ;
#2573=ORIENTED_EDGE ( 'NONE', *, *, #7, .T. ) ;
#2576=DIRECTION ( 'NONE',  ( -0.000000000000000000, 1.000000000000000000, -0.000000000000000000 ) ) ;
#2577=DIRECTION ( 'NONE',  ( 0.000000000000000000, 0.000000000000000000, -1.000000000000000000 ) ) ;
#2578=CARTESIAN_POINT ( 'NONE',  ( -23.15769640663937423, -133.1457019118818721, -48.00000000000002132 ) ) ;
#2579=CARTESIAN_POINT ( 'NONE',  ( -40.00000000000002842, -135.1457019118818721, 43.99999999999997158 ) ) ;
#2582=CIRCLE ( 'NONE', #4777, 4.000000000000000000 ) ;
#2584=ORIENTED_EDGE ( 'NONE', *, *, #3629, .T. ) ;
#2586=VERTEX_POINT ( 'NONE', #8877 ) ;
#2587=CARTESIAN_POINT ( 'NONE',  ( 53.40242741783141156, 52.77167129626698028, -30.00000000000000355 ) ) ;
#2593=AXIS2_PLACEMENT_3D ( 'NONE', #5648, #6444, #9694 ) ;
#2594=DIRECTION ( 'NONE',  ( 0.07334937666141724821, -0.9973063064792989652, -0.000000000000000000 ) ) ;
#2596=VERTEX_POINT ( 'NONE', #9531 ) ;
#2600=FACE_OUTER_BOUND ( 'NONE', #4884, .T. ) ;
#2601=FACE_OUTER_BOUND ( 'NONE', #5744, .T. ) ;
#2603=AXIS2_PLACEMENT_3D ( 'NONE', #8731, #7100, #9647 ) ;
#2605=CARTESIAN_POINT ( 'NONE',  ( -48.00000000000002132, -133.1457019118818721, -25.15769640663945950 ) ) ;
#2611=ORIENTED_EDGE ( 'NONE', *, *, #2371, .F. ) ;
#2614=DIRECTION ( 'NONE',  ( -6.982941293900105430E-16, 0.000000000000000000, 1.000000000000000000 ) ) ;
#2615=PLANE ( 'NONE',  #10186 ) ;
#2616=DIRECTION ( 'NONE',  ( 0.000000000000000000, -1.000000000000000000, 0.000000000000000000 ) ) ;
#2617=CARTESIAN_POINT ( 'NONE',  ( 0.000000000000000000, -133.1457019118818721, 25.15769640663938134 ) ) ;
#2619=CARTESIAN_POINT ( 'NONE',  ( 37.71464122736490054, -135.1457019118818721, -27.15769640663940265 ) ) ;
#2620=VECTOR ( 'NONE', #7443, 1000.000000000000000 ) ;
#2622=LINE ( 'NONE', #9897, #2410 ) ;
#2623=B_SPLINE_CURVE_WITH_KNOTS ( 'NONE', 3,
 ( #2619, #3368, #9730, #5842, #2456, #8021, #4003, #2403, #1612, #819, #4055, #9136, #2716, #346, #5897, #6856 ),
 .UNSPECIFIED., .F., .F.,
 ( 4, 2, 2, 2, 2, 2, 2, 4 ),
 ( 0.000000000000000000, 0.0003992569680943842936, 0.0007985139361887685873, 0.001197770904283152827, 0.001597027872377537175, 0.002395541808566243203, 0.002794798776660634924, 0.003194055744755026210 ),
 .UNSPECIFIED. ) ;
#2625=EDGE_CURVE ( 'NONE', #8577, #6600, #5559, .T. ) ;
#2626=ORIENTED_EDGE ( 'NONE', *, *, #9305, .F. ) ;
#2629=DIRECTION ( 'NONE',  ( 0.000000000000000000, -0.000000000000000000, -1.000000000000000000 ) ) ;
#2630=VERTEX_POINT ( 'NONE', #823 ) ;
#2631=CIRCLE ( 'NONE', #4821, 2.000000000000001776 ) ;
#2632=DIRECTION ( 'NONE',  ( -1.000000000000000000, 0.000000000000000000, 0.000000000000000000 ) ) ;
#2634=CARTESIAN_POINT ( 'NONE',  ( 39.99999999999998579, -135.1457019118818721, -40.00000000000002132 ) ) ;
#2635=LINE ( 'NONE', #2579, #9509 ) ;
#2640=DIRECTION ( 'NONE',  ( -0.000000000000000000, -0.000000000000000000, 1.000000000000000000 ) ) ;
#2641=ORIENTED_EDGE ( 'NONE', *, *, #3330, .F. ) ;
#2644=CARTESIAN_POINT ( 'NONE',  ( 4.856471286862176662, 145.0444252872335937, -30.00000000000000355 ) ) ;
#2646=AXIS2_PLACEMENT_3D ( 'NONE', #4728, #2297, #7074 ) ;
#2652=CARTESIAN_POINT ( 'NONE',  ( 25.15769640663938134, -133.1457019118818721, -27.15769640663941331 ) ) ;
#2654=EDGE_CURVE ( 'NONE', #1005, #4437, #6401, .T. ) ;
#2656=AXIS2_PLACEMENT_3D ( 'NONE', #10388, #6352, #5604 ) ;
#2657=EDGE_LOOP ( 'NONE', ( #1801, #3906 ) ) ;
#2660=CIRCLE ( 'NONE', #4019, 24.24539146688411861 ) ;
#2661=DIRECTION ( 'NONE',  ( 0.000000000000000000, 0.000000000000000000, 1.000000000000000000 ) ) ;
#2662=AXIS2_PLACEMENT_3D ( 'NONE', #351, #6805, #2776 ) ;
#2666=CARTESIAN_POINT ( 'NONE',  ( 17.97972049165455388, 37.08684478514406635, 30.00000000000000355 ) ) ;
#2667=LINE ( 'NONE', #6641, #1559 ) ;
#2669=EDGE_CURVE ( 'NONE', #1563, #389, #5043, .T. ) ;
#2672=ORIENTED_EDGE ( 'NONE', *, *, #9639, .F. ) ;
#2673=CARTESIAN_POINT ( 'NONE',  ( 42.22511195853866894, 17.84145331825995839, -30.00000000000000355 ) ) ;
#2675=CARTESIAN_POINT ( 'NONE',  ( -27.15769640663937778, -135.1457019118818721, -48.00000000000002132 ) ) ;
#2678=DIRECTION ( 'NONE',  ( 1.000000000000000000, 0.000000000000000000, 0.000000000000000000 ) ) ;
#2680=DIRECTION ( 'NONE',  ( -0.000000000000000000, 1.000000000000000000, -0.000000000000000000 ) ) ;
#2681=EDGE_CURVE ( 'NONE', #6001, #9740, #4395, .T. ) ;
#2682=EDGE_CURVE ( 'NONE', #8294, #3699, #9953, .T. ) ;
#2687=ORIENTED_EDGE ( 'NONE', *, *, #9950, .F. ) ;
#2691=CARTESIAN_POINT ( 'NONE',  ( -25.15769640663940621, -117.1457019118819005, 27.15769640663938489 ) ) ;
#2692=CARTESIAN_POINT ( 'NONE',  ( -48.00000000000002132, -133.1457019118818721, 27.15769640663938489 ) ) ;
#2693=DIRECTION ( 'NONE',  ( -0.9973063064792990762, -0.07334937666141726209, 0.000000000000000000 ) ) ;
#2694=CARTESIAN_POINT ( 'NONE',  ( 39.99999999999997158, -135.1457019118818721, 39.99999999999997868 ) ) ;
#2696=EDGE_CURVE ( 'NONE', #5111, #5490, #5902, .T. ) ;
#2697=DIRECTION ( 'NONE',  ( -0.000000000000000000, 1.000000000000000000, -0.000000000000000000 ) ) ;
#2698=VERTEX_POINT ( 'NONE', #7450 ) ;
#2700=CARTESIAN_POINT ( 'NONE',  ( 94.78677303995212355, -145.1457019118819005, -30.00000000000000355 ) ) ;
#2702=CARTESIAN_POINT ( 'NONE',  ( 4.856471286862175774, 152.5696653505793279, 30.00000000000000355 ) ) ;
#2704=ORIENTED_EDGE ( 'NONE', *, *, #9568, .T. ) ;
#2707=FACE_OUTER_BOUND ( 'NONE', #7118, .T. ) ;
#2708=EDGE_CURVE ( 'NONE', #8577, #1967, #248, .T. ) ;
#2710=EDGE_LOOP ( 'NONE', ( #9393, #4163, #9139, #4148 ) ) ;
#2712=FACE_OUTER_BOUND ( 'NONE', #796, .T. ) ;
#2713=FACE_OUTER_BOUND ( 'NONE', #2710, .T. ) ;
#2714=FACE_OUTER_BOUND ( 'NONE', #8892, .T. ) ;
#2715=DIRECTION ( 'NONE',  ( 0.000000000000000000, 0.000000000000000000, -1.000000000000000000 ) ) ;
#2716=CARTESIAN_POINT ( 'NONE',  ( 37.23009335863751801, -133.6763800654832153, -25.22473604584575924 ) ) ;
#2718=CARTESIAN_POINT ( 'NONE',  ( 39.99999999999997158, -135.1457019118818721, 35.99999999999999289 ) ) ;
#2722=EDGE_CURVE ( 'NONE', #10235, #991, #5056, .T. ) ;
#2723=VERTEX_POINT ( 'NONE', #2518 ) ;
#2725=AXIS2_PLACEMENT_3D ( 'NONE', #1412, #4640, #7088 ) ;
#2728=CARTESIAN_POINT ( 'NONE',  ( -25.15769640663940621, -133.1457019118818721, 27.15769640663938489 ) ) ;
#2730=ORIENTED_EDGE ( 'NONE', *, *, #4878, .F. ) ;
#2731=DIRECTION ( 'NONE',  ( -0.000000000000000000, 1.000000000000000000, 0.000000000000000000 ) ) ;
#2732=VERTEX_POINT ( 'NONE', #5800 ) ;
#2738=ADVANCED_FACE ( 'NONE', ( #5743, #1879 ), #1723, .F. ) ;
#2740=FACE_OUTER_BOUND ( 'NONE', #260, .T. ) ;
#2748=ORIENTED_EDGE ( 'NONE', *, *, #6572, .T. ) ;
#2753=ADVANCED_FACE ( 'NONE', ( #1828 ), #926, .T. ) ;
#2754=AXIS2_PLACEMENT_3D ( 'NONE', #8874, #9084, #8289 ) ;
#2755=CARTESIAN_POINT ( 'NONE',  ( 39.99999999999998579, -135.1457019118818721, -35.97500000000002274 ) ) ;
#2756=DIRECTION ( 'NONE',  ( -1.000000000000000000, -1.802741689055041147E-15, 0.000000000000000000 ) ) ;
#2759=ORIENTED_EDGE ( 'NONE', *, *, #332, .T. ) ;
#2761=ORIENTED_EDGE ( 'NONE', *, *, #259, .F. ) ;
#2765=CIRCLE ( 'NONE', #6833, 3.999999999999996447 ) ;
#2766=DIRECTION ( 'NONE',  ( 0.000000000000000000, 0.000000000000000000, 1.000000000000000000 ) ) ;
#2769=DIRECTION ( 'NONE',  ( -0.000000000000000000, 1.000000000000000000, -0.000000000000000000 ) ) ;
#2771=CARTESIAN_POINT ( 'NONE',  ( -38.19229777560033057, 37.08684478514405214, 12.50000000000000000 ) ) ;
#2776=DIRECTION ( 'NONE',  ( 0.000000000000000000, 0.000000000000000000, 1.000000000000000000 ) ) ;
#2777=AXIS2_PLACEMENT_3D ( 'NONE', #3046, #7085, #2199 ) ;
#2778=CARTESIAN_POINT ( 'NONE',  ( 37.71464122736488633, -135.1457019118818721, 27.15769640663938489 ) ) ;
#2780=CARTESIAN_POINT ( 'NONE',  ( 25.15769640663936357, -117.1457019118819005, 27.15769640663938489 ) ) ;
#2782=ORIENTED_EDGE ( 'NONE', *, *, #2264, .F. ) ;
#2783=CARTESIAN_POINT ( 'NONE',  ( 14.70649310359190309, 120.5696653505793705, -16.00000000000000711 ) ) ;
#2788=AXIS2_PLACEMENT_3D ( 'NONE', #4184, #7417, #3388 ) ;
#2790=LINE ( 'NONE', #4393, #5178 ) ;
#2792=LINE ( 'NONE', #10017, #2527 ) ;
#2793=CARTESIAN_POINT ( 'NONE',  ( -50.00000000000002842, -145.1457019118819005, 39.99999999999997868 ) ) ;
#2799=EDGE_LOOP ( 'NONE', ( #8482, #7532, #663 ) ) ;
#2801=CIRCLE ( 'NONE', #2983, 5.000000000000000888 ) ;
#2811=ADVANCED_FACE ( 'NONE', ( #6966 ), #7707, .T. ) ;
#2814=CIRCLE ( 'NONE', #2646, 1.999999999999998224 ) ;
#2815=VERTEX_POINT ( 'NONE', #5161 ) ;
#2820=CARTESIAN_POINT ( 'NONE',  ( 73.53765631853929108, 70.39106037767953694, 25.00000000000000000 ) ) ;
#2821=DIRECTION ( 'NONE',  ( 0.000000000000000000, 0.000000000000000000, 1.000000000000000000 ) ) ;
#2824=CARTESIAN_POINT ( 'NONE',  ( -23.48622939173161228, -144.8896666241527669, 3.853145670227867470 ) ) ;
#2825=ADVANCED_FACE ( 'NONE', ( #9353 ), #9403, .F. ) ;
#2830=CIRCLE ( 'NONE', #2497, 4.000000000000000000 ) ;
#2831=CARTESIAN_POINT ( 'NONE',  ( 27.15769640663935647, -135.1457019118818721, 2.654968395591742513E-14 ) ) ;
#2834=CARTESIAN_POINT ( 'NONE',  ( 37.23183231822027750, -133.8039134404564265, 25.26438245347419809 ) ) ;
#2837=ORIENTED_EDGE ( 'NONE', *, *, #7165, .T. ) ;
#2840=ORIENTED_EDGE ( 'NONE', *, *, #239, .F. ) ;
#2841=VECTOR ( 'NONE', #10131, 1000.000000000000000 ) ;
#2846=ORIENTED_EDGE ( 'NONE', *, *, #7542, .F. ) ;
#2853=DIRECTION ( 'NONE',  ( 1.000000000000000000, 0.000000000000000000, 0.000000000000000000 ) ) ;
#2857=CARTESIAN_POINT ( 'NONE',  ( -23.64290342185649152, -133.6308916829187297, -50.00000000000002132 ) ) ;
#2859=EDGE_CURVE ( 'NONE', #979, #6462, #1351, .T. ) ;
#2860=DIRECTION ( 'NONE',  ( -0.000000000000000000, -0.000000000000000000, 1.000000000000000000 ) ) ;
#2862=CYLINDRICAL_SURFACE ( 'NONE', #8176, 2.000000000000001776 ) ;
#2865=ORIENTED_EDGE ( 'NONE', *, *, #10056, .T. ) ;
#2866=CIRCLE ( 'NONE', #9658, 4.025000000000000355 ) ;
#2870=DIRECTION ( 'NONE',  ( 0.000000000000000000, 1.000000000000000000, -0.000000000000000000 ) ) ;
#2871=LINE ( 'NONE', #7699, #8487 ) ;
#2876=LINE ( 'NONE', #9082, #8908 ) ;
#2877=ORIENTED_EDGE ( 'NONE', *, *, #5082, .F. ) ;
#2879=FACE_OUTER_BOUND ( 'NONE', #7608, .T. ) ;
#2880=ADVANCED_FACE ( 'NONE', ( #2879 ), #9196, .F. ) ;
#2881=ORIENTED_EDGE ( 'NONE', *, *, #8505, .F. ) ;
#2887=DIRECTION ( 'NONE',  ( 0.000000000000000000, 0.000000000000000000, 1.000000000000000000 ) ) ;
#2888=EDGE_LOOP ( 'NONE', ( #7498, #7920, #2573, #7580, #7284, #6178, #5569, #1943 ) ) ;
#2889=AXIS2_PLACEMENT_3D ( 'NONE', #5445, #9542, #10284 ) ;
#2890=LINE ( 'NONE', #2783, #7318 ) ;
#2891=ORIENTED_EDGE ( 'NONE', *, *, #2033, .F. ) ;
#2892=ORIENTED_EDGE ( 'NONE', *, *, #7097, .T. ) ;
#2893=CARTESIAN_POINT ( 'NONE',  ( 73.53765631853929108, 70.39106037767955115, -30.00000000000000355 ) ) ;
#2894=VERTEX_POINT ( 'NONE', #400 ) ;
#2895=EDGE_CURVE ( 'NONE', #8447, #5933, #10098, .T. ) ;
#2898=CARTESIAN_POINT ( 'NONE',  ( 25.15769640663936002, -117.1457019118819005, -3.513494341946486113E-15 ) ) ;
#2900=EDGE_LOOP ( 'NONE', ( #1269, #8461, #5279, #9476, #2226, #8437, #9274, #10128, #6802, #7789, #10177, #7511, #3021, #189 ) ) ;
#2901=CARTESIAN_POINT ( 'NONE',  ( 27.15769640663936713, -135.1457019118818721, 25.15769640663938134 ) ) ;
#2906=AXIS2_PLACEMENT_3D ( 'NONE', #9156, #5073, #6771 ) ;
#2907=TOROIDAL_SURFACE ( 'NONE', #5277, 2.525240063345735475, 5.000000000000000000 ) ;
#2913=FACE_OUTER_BOUND ( 'NONE', #6832, .T. ) ;
#2917=CARTESIAN_POINT ( 'NONE',  ( 77.30044127146538813, 73.68369600860394542, -25.00000000000000355 ) ) ;
#2925=LINE ( 'NONE', #1232, #7082 ) ;
#2928=CARTESIAN_POINT ( 'NONE',  ( 23.15769640663936357, -117.1457019118819005, 27.15769640663938489 ) ) ;
#2929=VECTOR ( 'NONE', #1808, 1000.000000000000000 ) ;
#2932=CARTESIAN_POINT ( 'NONE',  ( 10.51964330236497602, 150.0000000000000000, -12.49999999999999289 ) ) ;
#2934=AXIS2_PLACEMENT_3D ( 'NONE', #1159, #5973, #4339 ) ;
#2938=DIRECTION ( 'NONE',  ( -1.000000000000000000, 0.000000000000000000, 0.000000000000000000 ) ) ;
#2939=DIRECTION ( 'NONE',  ( -1.000000000000000000, 0.000000000000000000, 0.000000000000000000 ) ) ;
#2942=DIRECTION ( 'NONE',  ( -1.000000000000000000, 0.000000000000000000, 0.000000000000000000 ) ) ;
#2945=EDGE_CURVE ( 'NONE', #7279, #5671, #5627, .T. ) ;
#2951=CIRCLE ( 'NONE', #9388, 4.999999999999997335 ) ;
#2957=CARTESIAN_POINT ( 'NONE',  ( -18.34874108452141073, -140.1746510883711778, 49.99999999999997868 ) ) ;
#2964=EDGE_CURVE ( 'NONE', #4912, #6120, #330, .T. ) ;
#2966=FACE_OUTER_BOUND ( 'NONE', #6308, .T. ) ;
#2968=CARTESIAN_POINT ( 'NONE',  ( 80.08610854271792334, 54.73418909528891874, -30.00000000000000355 ) ) ;
#2969=ORIENTED_EDGE ( 'NONE', *, *, #5288, .F. ) ;
#2970=CARTESIAN_POINT ( 'NONE',  ( -50.00000000000002132, -135.0799149511624364, 25.93998375192767014 ) ) ;
#2971=DIRECTION ( 'NONE',  ( 0.000000000000000000, 0.000000000000000000, -1.000000000000000000 ) ) ;
#2973=EDGE_LOOP ( 'NONE', ( #4647, #2422, #143, #6227 ) ) ;
#2974=VERTEX_POINT ( 'NONE', #9780 ) ;
#2977=ORIENTED_EDGE ( 'NONE', *, *, #8446, .T. ) ;
#2978=CARTESIAN_POINT ( 'NONE',  ( -50.00000000000001421, -135.1457019118818721, -26.62179802177720944 ) ) ;
#2980=DIRECTION ( 'NONE',  ( 1.000000000000000000, -0.000000000000000000, -0.000000000000000000 ) ) ;
#2983=AXIS2_PLACEMENT_3D ( 'NONE', #7778, #9371, #6986 ) ;
#2985=AXIS2_PLACEMENT_3D ( 'NONE', #297, #3520, #6749 ) ;
#2986=EDGE_LOOP ( 'NONE', ( #4253, #1385, #9664, #1927 ) ) ;
#2987=CARTESIAN_POINT ( 'NONE',  ( -27.15769640663940976, -133.1457019118818721, 27.15769640663938489 ) ) ;
#2988=CIRCLE ( 'NONE', #4841, 2.000000000000001776 ) ;
#2991=EDGE_LOOP ( 'NONE', ( #5729, #2029, #9643, #7770 ) ) ;
#2998=EDGE_LOOP ( 'NONE', ( #7937, #7982, #10342, #4440 ) ) ;
#3005=VECTOR ( 'NONE', #2507, 1000.000000000000000 ) ;
#3006=ORIENTED_EDGE ( 'NONE', *, *, #4724, .T. ) ;
#3010=ORIENTED_EDGE ( 'NONE', *, *, #5727, .T. ) ;
#3014=DIRECTION ( 'NONE',  ( 0.000000000000000000, 0.000000000000000000, -1.000000000000000000 ) ) ;
#3015=DIRECTION ( 'NONE',  ( -0.000000000000000000, 1.000000000000000000, -0.000000000000000000 ) ) ;
#3016=FACE_OUTER_BOUND ( 'NONE', #10476, .T. ) ;
#3017=DIRECTION ( 'NONE',  ( 0.07334937666141726209, -0.9973063064792991872, 0.000000000000000000 ) ) ;
#3020=LINE ( 'NONE', #7895, #1802 ) ;
#3021=ORIENTED_EDGE ( 'NONE', *, *, #1874, .T. ) ;
#3023=AXIS2_PLACEMENT_3D ( 'NONE', #480, #7583, #5927 ) ;
#3024=EDGE_CURVE ( 'NONE', #6270, #8983, #6475, .T. ) ;
#3026=DIRECTION ( 'NONE',  ( 0.000000000000000000, 0.000000000000000000, -1.000000000000000000 ) ) ;
#3029=ORIENTED_EDGE ( 'NONE', *, *, #5409, .F. ) ;
#3031=VERTEX_POINT ( 'NONE', #8117 ) ;
#3033=ORIENTED_EDGE ( 'NONE', *, *, #3401, .F. ) ;
#3034=CARTESIAN_POINT ( 'NONE',  ( -50.00000000000001421, -134.8487302617674857, -25.28853996896960510 ) ) ;
#3035=DIRECTION ( 'NONE',  ( 0.000000000000000000, 0.000000000000000000, -1.000000000000000000 ) ) ;
#3036=CARTESIAN_POINT ( 'NONE',  ( -23.15769640663937423, -115.1457019118818863, -50.00000000000002132 ) ) ;
#3038=CARTESIAN_POINT ( 'NONE',  ( 39.99999999999998579, -135.1457019118818721, -36.00000000000002842 ) ) ;
#3040=AXIS2_PLACEMENT_3D ( 'NONE', #230, #3454, #2661 ) ;
#3043=ORIENTED_EDGE ( 'NONE', *, *, #251, .T. ) ;
#3044=DIRECTION ( 'NONE',  ( -1.396588258780021135E-16, 0.000000000000000000, 1.000000000000000000 ) ) ;
#3046=CARTESIAN_POINT ( 'NONE',  ( 4.856471286862175774, 147.5696653505793279, 25.00000000000000000 ) ) ;
#3048=ORIENTED_EDGE ( 'NONE', *, *, #7748, .T. ) ;
#3049=FACE_OUTER_BOUND ( 'NONE', #9259, .T. ) ;
#3051=ADVANCED_FACE ( 'NONE', ( #2707 ), #9177, .F. ) ;
#3054=VERTEX_POINT ( 'NONE', #1914 ) ;
#3055=ORIENTED_EDGE ( 'NONE', *, *, #8061, .F. ) ;
#3057=CARTESIAN_POINT ( 'NONE',  ( 27.15769640663938489, -115.1457019118818863, -25.15769640663940621 ) ) ;
#3059=DIRECTION ( 'NONE',  ( 0.000000000000000000, 0.000000000000000000, 1.000000000000000000 ) ) ;
#3064=EDGE_CURVE ( 'NONE', #732, #1563, #6847, .T. ) ;
#3067=AXIS2_PLACEMENT_3D ( 'NONE', #7046, #2326, #9649 ) ;
#3069=CYLINDRICAL_SURFACE ( 'NONE', #6576, 1.999999999999998224 ) ;
#3070=DIRECTION ( 'NONE',  ( -0.000000000000000000, 1.000000000000000000, -0.000000000000000000 ) ) ;
#3072=CARTESIAN_POINT ( 'NONE',  ( 42.22511195853866894, 17.84145331825995839, -25.00000000000000000 ) ) ;
#3073=AXIS2_PLACEMENT_3D ( 'NONE', #3766, #4755, #7844 ) ;
#3074=CYLINDRICAL_SURFACE ( 'NONE', #8374, 2.000000000000001776 ) ;
#3075=CIRCLE ( 'NONE', #8997, 2.000000000000001776 ) ;
#3076=ORIENTED_EDGE ( 'NONE', *, *, #10298, .T. ) ;
#3078=ORIENTED_EDGE ( 'NONE', *, *, #6096, .F. ) ;
#3079=EDGE_CURVE ( 'NONE', #6094, #2732, #3617, .T. ) ;
#3080=ADVANCED_FACE ( 'NONE', ( #3510 ), #284, .T. ) ;
#3082=VECTOR ( 'NONE', #1634, 1000.000000000000000 ) ;
#3087=LINE ( 'NONE', #751, #8740 ) ;
#3089=CARTESIAN_POINT ( 'NONE',  ( 4.856471286862175774, 152.5696653505793279, 30.00000000000000355 ) ) ;
#3094=FACE_OUTER_BOUND ( 'NONE', #2538, .T. ) ;
#3096=EDGE_CURVE ( 'NONE', #9582, #1800, #2193, .T. ) ;
#3098=CYLINDRICAL_SURFACE ( 'NONE', #9731, 5.000000000000001776 ) ;
#3099=SPHERICAL_SURFACE ( 'NONE', #9588, 2.000000000000000000 ) ;
#3100=EDGE_LOOP ( 'NONE', ( #366, #6420, #327, #9360 ) ) ;
#3104=ORIENTED_EDGE ( 'NONE', *, *, #2443, .F. ) ;
#3106=ORIENTED_EDGE ( 'NONE', *, *, #4462, .T. ) ;
#3110=( NAMED_UNIT ( * ) PLANE_ANGLE_UNIT ( ) SI_UNIT ( $, .RADIAN. ) );
#3116=ORIENTED_EDGE ( 'NONE', *, *, #746, .T. ) ;
#3118=AXIS2_PLACEMENT_3D ( 'NONE', #7985, #10333, #3014 ) ;
#3119=DIRECTION ( 'NONE',  ( -0.000000000000000000, 1.000000000000000000, -0.000000000000000000 ) ) ;
#3120=ORIENTED_EDGE ( 'NONE', *, *, #4037, .T. ) ;
#3121=CARTESIAN_POINT ( 'NONE',  ( 14.70649310359190309, 120.5696653505793705, -20.00000000000000711 ) ) ;
#3130=ORIENTED_EDGE ( 'NONE', *, *, #8952, .F. ) ;
#3134=CARTESIAN_POINT ( 'NONE',  ( 26.62179802177712062, -135.1457019118818721, 49.99999999999997868 ) ) ;
#3135=AXIS2_PLACEMENT_3D ( 'NONE', #1575, #4017, #1478 ) ;
#3136=CARTESIAN_POINT ( 'NONE',  ( -26.62179802177712773, -135.1457019118818721, -50.00000000000002132 ) ) ;
#3138=EDGE_CURVE ( 'NONE', #6261, #10221, #7463, .T. ) ;
#3139=EDGE_CURVE ( 'NONE', #7930, #7422, #1740, .T. ) ;
#3140=EDGE_CURVE ( 'NONE', #4400, #5439, #1847, .T. ) ;
#3144=VECTOR ( 'NONE', #3534, 1000.000000000000000 ) ;
#3147=DIRECTION ( 'NONE',  ( -9.776117811460147207E-16, 0.000000000000000000, 1.000000000000000000 ) ) ;
#3149=EDGE_CURVE ( 'NONE', #4871, #4567, #3717, .T. ) ;
#3152=ORIENTED_EDGE ( 'NONE', *, *, #10202, .F. ) ;
#3153=CARTESIAN_POINT ( 'NONE',  ( 14.70649310359190309, 120.5696653505793705, -16.00000000000000711 ) ) ;
#3158=ORIENTED_EDGE ( 'NONE', *, *, #2304, .F. ) ;
#3162=DIRECTION ( 'NONE',  ( 0.7525569905852184105, 0.6585271261848820723, 0.000000000000000000 ) ) ;
#3164=EDGE_LOOP ( 'NONE', ( #8959, #7461, #115, #1551 ) ) ;
#3165=SPHERICAL_SURFACE ( 'NONE', #3573, 2.000000000000000000 ) ;
#3167=EDGE_CURVE ( 'NONE', #8341, #5589, #9757, .T. ) ;
#3169=CIRCLE ( 'NONE', #4692, 3.999999999999989786 ) ;
#3170=LINE ( 'NONE', #7155, #7907 ) ;
#3171=AXIS2_PLACEMENT_3D ( 'NONE', #4196, #5035, #4978 ) ;
#3173=DIRECTION ( 'NONE',  ( -0.000000000000000000, 1.000000000000000000, -0.000000000000000000 ) ) ;
#3174=CARTESIAN_POINT ( 'NONE',  ( 27.15769640663938489, -115.1457019118818863, -27.15769640663940976 ) ) ;
#3180=VERTEX_POINT ( 'NONE', #2431 ) ;
#3183=CIRCLE ( 'NONE', #1506, 3.999999999999989786 ) ;
#3185=CARTESIAN_POINT ( 'NONE',  ( -23.15769640663939199, -115.1457019118818863, -27.15769640663944173 ) ) ;
#3186=CARTESIAN_POINT ( 'NONE',  ( -2.293506896408101348, 147.5696653505793279, 25.00000000000000000 ) ) ;
#3188=CARTESIAN_POINT ( 'NONE',  ( -25.15769640663940976, -115.1457019118818863, -1.756747170973246291E-14 ) ) ;
#3191=EDGE_LOOP ( 'NONE', ( #3211, #1361 ) ) ;
#3195=ADVANCED_FACE ( 'NONE', ( #5707 ), #8950, .T. ) ;
#3197=DIRECTION ( 'NONE',  ( -0.000000000000000000, 1.000000000000000000, -0.000000000000000000 ) ) ;
#3198=VECTOR ( 'NONE', #9157, 1000.000000000000000 ) ;
#3200=LINE ( 'NONE', #5737, #6538 ) ;
#3201=ORIENTED_EDGE ( 'NONE', *, *, #516, .T. ) ;
#3206=EDGE_CURVE ( 'NONE', #7078, #3286, #5572, .T. ) ;
#3209=AXIS2_PLACEMENT_3D ( 'NONE', #4745, #9538, #6184 ) ;
#3210=ORIENTED_EDGE ( 'NONE', *, *, #6310, .F. ) ;
#3211=ORIENTED_EDGE ( 'NONE', *, *, #7068, .F. ) ;
#3212=LINE ( 'NONE', #40, #2148 ) ;
#3213=DIRECTION ( 'NONE',  ( 0.000000000000000000, 0.000000000000000000, -1.000000000000000000 ) ) ;
#3216=DIRECTION ( 'NONE',  ( 0.000000000000000000, 0.000000000000000000, 1.000000000000000000 ) ) ;
#3217=EDGE_LOOP ( 'NONE', ( #9090, #1853, #7877, #9505 ) ) ;
#3218=EDGE_CURVE ( 'NONE', #9452, #7162, #6881, .T. ) ;
#3219=DIRECTION ( 'NONE',  ( 0.000000000000000000, -1.000000000000000000, 0.000000000000000000 ) ) ;
#3222=CARTESIAN_POINT ( 'NONE',  ( -40.00000000000001421, -145.1457019118819005, -40.00000000000002132 ) ) ;
#3223=DIRECTION ( 'NONE',  ( -0.000000000000000000, -0.000000000000000000, 1.000000000000000000 ) ) ;
#3224=LINE ( 'NONE', #7999, #9195 ) ;
#3227=CARTESIAN_POINT ( 'NONE',  ( -16.29350689640809691, -115.1457019118818863, 30.31717237747080773 ) ) ;
#3229=EDGE_LOOP ( 'NONE', ( #9255, #10422, #1280, #2204 ) ) ;
#3230=CIRCLE ( 'NONE', #9153, 2.000000000000001776 ) ;
#3231=ORIENTED_EDGE ( 'NONE', *, *, #8582, .F. ) ;
#3232=ORIENTED_EDGE ( 'NONE', *, *, #2264, .T. ) ;
#3236=VECTOR ( 'NONE', #4886, 1000.000000000000000 ) ;
#3244=ORIENTED_EDGE ( 'NONE', *, *, #5409, .T. ) ;
#3245=ORIENTED_EDGE ( 'NONE', *, *, #3656, .T. ) ;
#3246=DIRECTION ( 'NONE',  ( -1.387778780781445676E-16, 0.000000000000000000, 1.000000000000000000 ) ) ;
#3250=LINE ( 'NONE', #3366, #2620 ) ;
#3251=EDGE_CURVE ( 'NONE', #4567, #10220, #5179, .T. ) ;
#3252=FACE_OUTER_BOUND ( 'NONE', #2236, .T. ) ;
#3253=ORIENTED_EDGE ( 'NONE', *, *, #5977, .T. ) ;
#3254=DIRECTION ( 'NONE',  ( -0.000000000000000000, 1.000000000000000000, -0.000000000000000000 ) ) ;
#3256=ORIENTED_EDGE ( 'NONE', *, *, #5144, .F. ) ;
#3259=B_SPLINE_CURVE_WITH_KNOTS ( 'NONE', 3,
 ( #3136, #9668, #9620, #8808, #1549, #4772, #6998, #2857, #2010, #1217 ),
 .UNSPECIFIED., .F., .F.,
 ( 4, 2, 2, 2, 4 ),
 ( 0.000000000000000000, 0.001023740819106960624, 0.002047481638213921248, 0.003071222457320881873, 0.004094963276427842497 ),
 .UNSPECIFIED. ) ;
#3261=VERTEX_POINT ( 'NONE', #6133 ) ;
#3263=CYLINDRICAL_SURFACE ( 'NONE', #8072, 7.525240063345735919 ) ;
#3264=PLANE ( 'NONE',  #4794 ) ;
#3266=EDGE_CURVE ( 'NONE', #2723, #2339, #2792, .T. ) ;
#3267=DIRECTION ( 'NONE',  ( -1.000000000000000000, -0.000000000000000000, -0.000000000000000000 ) ) ;
#3272=EDGE_LOOP ( 'NONE', ( #4539, #2892, #3576, #2047 ) ) ;
#3275=ORIENTED_EDGE ( 'NONE', *, *, #9064, .F. ) ;
#3276=CARTESIAN_POINT ( 'NONE',  ( 0.000000000000000000, -145.1457019118819005, -50.00000000000002132 ) ) ;
#3281=EDGE_CURVE ( 'NONE', #5030, #7304, #6592, .T. ) ;
#3282=CARTESIAN_POINT ( 'NONE',  ( -38.19229777560033057, -43.28483205141633761, 12.50000000000000000 ) ) ;
#3284=AXIS2_PLACEMENT_3D ( 'NONE', #456, #6922, #10157 ) ;
#3285=ORIENTED_EDGE ( 'NONE', *, *, #871, .T. ) ;
#3286=VERTEX_POINT ( 'NONE', #10121 ) ;
#3290=FACE_OUTER_BOUND ( 'NONE', #9902, .T. ) ;
#3295=ORIENTED_EDGE ( 'NONE', *, *, #5202, .T. ) ;
#3298=EDGE_CURVE ( 'NONE', #415, #6001, #7676, .T. ) ;
#3300=AXIS2_PLACEMENT_3D ( 'NONE', #9497, #9707, #4809 ) ;
#3303=DIRECTION ( 'NONE',  ( 0.000000000000000000, 0.000000000000000000, 1.000000000000000000 ) ) ;
#3304=CARTESIAN_POINT ( 'NONE',  ( -2.293506896408097795, 152.5696653505793279, 30.00000000000000355 ) ) ;
#3306=DIRECTION ( 'NONE',  ( 1.000000000000000000, 0.000000000000000000, 0.000000000000000000 ) ) ;
#3307=ORIENTED_EDGE ( 'NONE', *, *, #5332, .T. ) ;
#3308=DIRECTION ( 'NONE',  ( -0.000000000000000000, 1.000000000000000000, -0.000000000000000000 ) ) ;
#3310=ORIENTED_EDGE ( 'NONE', *, *, #7153, .T. ) ;
#3311=CIRCLE ( 'NONE', #1794, 1.999999999999998224 ) ;
#3314=EDGE_LOOP ( 'NONE', ( #2465, #74, #9401, #6210 ) ) ;
#3315=CONICAL_SURFACE ( 'NONE', #9062, 4.025000000000000355, 0.7853981633975870569 ) ;
#3319=CARTESIAN_POINT ( 'NONE',  ( -18.34874108452141783, -140.1746510883711778, -7.212905963064413228 ) ) ;
#3321=CIRCLE ( 'NONE', #953, 5.000000000000004441 ) ;
#3322=CARTESIAN_POINT ( 'NONE',  ( -26.62179802177716326, -135.1457019118818721, 49.99999999999997868 ) ) ;
#3325=AXIS2_PLACEMENT_3D ( 'NONE', #10406, #7175, #6160 ) ;
#3326=VERTEX_POINT ( 'NONE', #2106 ) ;
#3330=EDGE_CURVE ( 'NONE', #3785, #7273, #2866, .T. ) ;
#3331=ADVANCED_FACE ( 'NONE', ( #7517 ), #9972, .F. ) ;
#3332=ORIENTED_EDGE ( 'NONE', *, *, #8736, .T. ) ;
#3337=AXIS2_PLACEMENT_3D ( 'NONE', #1882, #10102, #9957 ) ;
#3339=LINE ( 'NONE', #7465, #71 ) ;
#3340=CARTESIAN_POINT ( 'NONE',  ( 53.40242741783141156, 52.77167129626698028, -25.00000000000000355 ) ) ;
#3345=AXIS2_PLACEMENT_3D ( 'NONE', #175, #120, #3354 ) ;
#3346=ADVANCED_FACE ( 'NONE', ( #3548 ), #9215, .F. ) ;
#3350=CARTESIAN_POINT ( 'NONE',  ( -48.00000000000002132, -135.1457019118818721, -23.15769640663945594 ) ) ;
#3354=DIRECTION ( 'NONE',  ( 0.000000000000000000, 0.000000000000000000, 1.000000000000000000 ) ) ;
#3356=DIRECTION ( 'NONE',  ( 0.000000000000000000, 0.000000000000000000, 1.000000000000000000 ) ) ;
#3359=VERTEX_POINT ( 'NONE', #2957 ) ;
#3364=CARTESIAN_POINT ( 'NONE',  ( 53.40242741783141156, 52.77167129626698028, 30.00000000000000355 ) ) ;
#3366=CARTESIAN_POINT ( 'NONE',  ( 2.108096605167896559E-14, -133.1457019118818721, -25.15769640663943107 ) ) ;
#3367=EDGE_CURVE ( 'NONE', #8668, #4826, #1855, .T. ) ;
#3368=CARTESIAN_POINT ( 'NONE',  ( 37.65645052921861691, -135.1457019118819289, -27.03605397352983175 ) ) ;
#3371=ORIENTED_EDGE ( 'NONE', *, *, #9788, .F. ) ;
#3372=DIRECTION ( 'NONE',  ( -1.000000000000000000, -0.000000000000000000, -0.000000000000000000 ) ) ;
#3373=ORIENTED_EDGE ( 'NONE', *, *, #2280, .T. ) ;
#3374=VECTOR ( 'NONE', #553, 1000.000000000000000 ) ;
#3375=DIRECTION ( 'NONE',  ( 0.000000000000000000, -1.000000000000000000, 0.000000000000000000 ) ) ;
#3379=LINE ( 'NONE', #1038, #1051 ) ;
#3381=VERTEX_POINT ( 'NONE', #2366 ) ;
#3385=CARTESIAN_POINT ( 'NONE',  ( 18.34874108452142494, -140.1746510883711778, 49.99999999999997868 ) ) ;
#3388=DIRECTION ( 'NONE',  ( -8.379529552680124346E-16, 0.000000000000000000, 1.000000000000000000 ) ) ;
#3395=CARTESIAN_POINT ( 'NONE',  ( -2.293506896408097795, 37.08684478514406635, 30.00000000000000355 ) ) ;
#3399=ADVANCED_FACE ( 'NONE', ( #7886 ), #8676, .F. ) ;
#3401=EDGE_CURVE ( 'NONE', #4076, #7523, #2364, .T. ) ;
#3402=EDGE_CURVE ( 'NONE', #3742, #3545, #3724, .T. ) ;
#3404=CARTESIAN_POINT ( 'NONE',  ( -25.15769640663940621, -115.1457019118818863, 23.15769640663938134 ) ) ;
#3408=LINE ( 'NONE', #7382, #10297 ) ;
#3409=DIRECTION ( 'NONE',  ( 0.000000000000000000, 0.000000000000000000, 1.000000000000000000 ) ) ;
#3417=CARTESIAN_POINT ( 'NONE',  ( 42.22511195853867605, 17.84145331825995839, 30.00000000000000355 ) ) ;
#3423=CIRCLE ( 'NONE', #540, 2.000000000000001776 ) ;
#3425=CARTESIAN_POINT ( 'NONE',  ( 59.99999999999999289, -135.1457019118818721, -40.00000000000000000 ) ) ;
#3426=DIRECTION ( 'NONE',  ( 0.000000000000000000, -1.000000000000000000, 0.000000000000000000 ) ) ;
#3427=CARTESIAN_POINT ( 'NONE',  ( 99.80027788547049283, -145.1457019118819005, -24.99999999999998934 ) ) ;
#3432=ADVANCED_FACE ( 'NONE', ( #7099 ), #1476, .F. ) ;
#3434=FACE_OUTER_BOUND ( 'NONE', #8159, .T. ) ;
#3435=CARTESIAN_POINT ( 'NONE',  ( -27.15769640663939555, -133.1457019118818721, -25.15769640663944173 ) ) ;
#3438=DIRECTION ( 'NONE',  ( -1.000000000000000000, -0.000000000000000000, -0.000000000000000000 ) ) ;
#3439=DIRECTION ( 'NONE',  ( 0.000000000000000000, 0.000000000000000000, 1.000000000000000000 ) ) ;
#3440=MANIFOLD_SOLID_BREP ( 'Cut-Extrude11', #4359 ) ;
#3442=ORIENTED_EDGE ( 'NONE', *, *, #3993, .F. ) ;
#3447=DIRECTION ( 'NONE',  ( 0.000000000000000000, 0.000000000000000000, 1.000000000000000000 ) ) ;
#3449=CIRCLE ( 'NONE', #2436, 4.000000000000000000 ) ;
#3453=VERTEX_POINT ( 'NONE', #10226 ) ;
#3454=DIRECTION ( 'NONE',  ( -1.000000000000000000, 0.000000000000000000, 0.000000000000000000 ) ) ;
#3456=EDGE_LOOP ( 'NONE', ( #2128, #9966, #6278, #6714 ) ) ;
#3458=ORIENTED_EDGE ( 'NONE', *, *, #1491, .T. ) ;
#3459=EDGE_CURVE ( 'NONE', #1518, #732, #575, .T. ) ;
#3460=DIRECTION ( 'NONE',  ( 0.000000000000000000, 1.000000000000000000, 0.000000000000000000 ) ) ;
#3462=PLANE ( 'NONE',  #2048 ) ;
#3463=ADVANCED_FACE ( 'NONE', ( #5693 ), #8988, .F. ) ;
#3464=LINE ( 'NONE', #2666, #8051 ) ;
#3465=LINE ( 'NONE', #1921, #6992 ) ;
#3467=AXIS2_PLACEMENT_3D ( 'NONE', #9867, #8152, #3439 ) ;
#3469=CARTESIAN_POINT ( 'NONE',  ( -40.00000000000002842, -135.1457019118818721, 44.02499999999997726 ) ) ;
#3477=CARTESIAN_POINT ( 'NONE',  ( 37.22759939293836595, -133.1457019118818721, 25.15769640663938134 ) ) ;
#3479=DIRECTION ( 'NONE',  ( 0.000000000000000000, -1.000000000000000000, 0.000000000000000000 ) ) ;
#3480=CARTESIAN_POINT ( 'NONE',  ( -2.293506896408097795, 147.5696653505793279, -30.00000000000000355 ) ) ;
#3483=CIRCLE ( 'NONE', #3995, 2.000000000000001776 ) ;
#3485=ORIENTED_EDGE ( 'NONE', *, *, #2669, .F. ) ;
#3493=FACE_OUTER_BOUND ( 'NONE', #5123, .T. ) ;
#3497=AXIS2_PLACEMENT_3D ( 'NONE', #7840, #2115, #4658 ) ;
#3498=EDGE_CURVE ( 'NONE', #996, #6001, #1303, .T. ) ;
#3499=AXIS2_PLACEMENT_3D ( 'NONE', #2370, #3017, #4800 ) ;
#3501=FACE_OUTER_BOUND ( 'NONE', #1979, .T. ) ;
#3503=LINE ( 'NONE', #2702, #6141 ) ;
#3504=CARTESIAN_POINT ( 'NONE',  ( 49.99999999999997158, -145.1457019118819005, 39.99999999999997868 ) ) ;
#3505=VECTOR ( 'NONE', #8202, 1000.000000000000000 ) ;
#3506=ORIENTED_EDGE ( 'NONE', *, *, #3064, .T. ) ;
#3508=VERTEX_POINT ( 'NONE', #1572 ) ;
#3509=STYLED_ITEM('',(#10497),#3440);
#3510=FACE_OUTER_BOUND ( 'NONE', #7003, .T. ) ;
#3513=VERTEX_POINT ( 'NONE', #4221 ) ;
#3515=CARTESIAN_POINT ( 'NONE',  ( 27.15769640663937068, -135.1457019118818721, 47.99999999999997868 ) ) ;
#3516=VECTOR ( 'NONE', #7691, 1000.000000000000000 ) ;
#3517=FACE_OUTER_BOUND ( 'NONE', #10362, .T. ) ;
#3520=DIRECTION ( 'NONE',  ( -0.000000000000000000, 1.000000000000000000, -0.000000000000000000 ) ) ;
#3524=EDGE_CURVE ( 'NONE', #2357, #8114, #4355, .T. ) ;
#3525=ORIENTED_EDGE ( 'NONE', *, *, #4374, .F. ) ;
#3528=ORIENTED_EDGE ( 'NONE', *, *, #4829, .T. ) ;
#3532=CARTESIAN_POINT ( 'NONE',  ( 25.15769640663938844, -117.1457019118819005, -50.00000000000002132 ) ) ;
#3534=DIRECTION ( 'NONE',  ( -0.000000000000000000, -0.000000000000000000, -1.000000000000000000 ) ) ;
#3536=EDGE_LOOP ( 'NONE', ( #6504, #5691, #8029 ) ) ;
#3537=DIRECTION ( 'NONE',  ( -1.000000000000000000, -0.000000000000000000, 0.000000000000000000 ) ) ;
#3538=EDGE_CURVE ( 'NONE', #5630, #6595, #7293, .T. ) ;
#3539=ADVANCED_FACE ( 'NONE', ( #773 ), #5593, .F. ) ;
#3540=EDGE_CURVE ( 'NONE', #6595, #8048, #3212, .T. ) ;
#3542=ORIENTED_EDGE ( 'NONE', *, *, #9304, .F. ) ;
#3543=FACE_OUTER_BOUND ( 'NONE', #3456, .T. ) ;
#3545=VERTEX_POINT ( 'NONE', #7246 ) ;
#3548=FACE_OUTER_BOUND ( 'NONE', #4416, .T. ) ;
#3549=DIRECTION ( 'NONE',  ( -1.000000000000000000, 0.000000000000000000, 0.000000000000000000 ) ) ;
#3553=ADVANCED_FACE ( 'NONE', ( #6439 ), #3263, .T. ) ;
#3556=CARTESIAN_POINT ( 'NONE',  ( 0.000000000000000000, -115.1457019118818863, 23.15769640663938134 ) ) ;
#3559=CARTESIAN_POINT ( 'NONE',  ( -50.00000000000001421, -134.0910007290637509, 24.15108826162072120 ) ) ;
#3561=VERTEX_POINT ( 'NONE', #6920 ) ;
#3564=ORIENTED_EDGE ( 'NONE', *, *, #10042, .T. ) ;
#3566=EDGE_CURVE ( 'NONE', #5617, #2069, #403, .T. ) ;
#3568=CARTESIAN_POINT ( 'NONE',  ( 0.000000000000000000, -117.1457019118819005, 25.15769640663938134 ) ) ;
#3569=DIRECTION ( 'NONE',  ( -0.000000000000000000, -1.000000000000000000, 0.000000000000000000 ) ) ;
#3570=DIRECTION ( 'NONE',  ( -1.000000000000000000, 0.000000000000000000, 0.000000000000000000 ) ) ;
#3573=AXIS2_PLACEMENT_3D ( 'NONE', #2273, #1425, #10335 ) ;
#3574=ORIENTED_EDGE ( 'NONE', *, *, #8155, .F. ) ;
#3576=ORIENTED_EDGE ( 'NONE', *, *, #3459, .F. ) ;
#3578=VECTOR ( 'NONE', #4263, 1000.000000000000000 ) ;
#3579=LINE ( 'NONE', #3532, #5697 ) ;
#3580=LINE ( 'NONE', #253, #5644 ) ;
#3581=DIRECTION ( 'NONE',  ( -0.000000000000000000, 1.000000000000000000, -0.000000000000000000 ) ) ;
#3582=DIRECTION ( 'NONE',  ( 0.000000000000000000, 1.000000000000000000, 0.000000000000000000 ) ) ;
#3587=VERTEX_POINT ( 'NONE', #7659 ) ;
#3590=AXIS2_PLACEMENT_3D ( 'NONE', #3610, #6144, #433 ) ;
#3593=FACE_OUTER_BOUND ( 'NONE', #4251, .T. ) ;
#3594=EDGE_CURVE ( 'NONE', #979, #3261, #6064, .T. ) ;
#3601=VECTOR ( 'NONE', #4649, 1000.000000000000000 ) ;
#3602=DIRECTION ( 'NONE',  ( 1.000000000000000000, 0.000000000000000000, 0.000000000000000000 ) ) ;
#3603=VECTOR ( 'NONE', #4067, 1000.000000000000000 ) ;
#3605=EDGE_LOOP ( 'NONE', ( #6326, #5462, #695, #8763 ) ) ;
#3606=ADVANCED_FACE ( 'NONE', ( #2036, #252, #5263 ), #10003, .F. ) ;
#3608=AXIS2_PLACEMENT_3D ( 'NONE', #4474, #451, #2030 ) ;
#3610=CARTESIAN_POINT ( 'NONE',  ( 14.70649310359190309, 80.56966535057935630, 20.00000000000000711 ) ) ;
#3611=EDGE_CURVE ( 'NONE', #6531, #7774, #2660, .T. ) ;
#3613=LINE ( 'NONE', #436, #1316 ) ;
#3614=EDGE_LOOP ( 'NONE', ( #4842, #10369, #3076, #10449 ) ) ;
#3615=AXIS2_PLACEMENT_3D ( 'NONE', #5348, #3718, #9334 ) ;
#3617=LINE ( 'NONE', #9286, #6084 ) ;
#3619=ORIENTED_EDGE ( 'NONE', *, *, #5880, .T. ) ;
#3622=CIRCLE ( 'NONE', #2603, 7.525240063345735031 ) ;
#3623=FACE_OUTER_BOUND ( 'NONE', #2986, .T. ) ;
#3629=EDGE_CURVE ( 'NONE', #4419, #1304, #4379, .T. ) ;
#3630=CIRCLE ( 'NONE', #4475, 2.000000000000001776 ) ;
#3633=VECTOR ( 'NONE', #2402, 1000.000000000000000 ) ;
#3635=CARTESIAN_POINT ( 'NONE',  ( 37.22759939293837306, -133.2806661801596420, 25.15769640663938489 ) ) ;
#3636=FACE_OUTER_BOUND ( 'NONE', #4430, .T. ) ;
#3639=DIRECTION ( 'NONE',  ( 0.000000000000000000, 0.000000000000000000, -1.000000000000000000 ) ) ;
#3640=ORIENTED_EDGE ( 'NONE', *, *, #6886, .F. ) ;
#3644=CIRCLE ( 'NONE', #4984, 2.000000000000001776 ) ;
#3645=LINE ( 'NONE', #9317, #1810 ) ;
#3646=EDGE_LOOP ( 'NONE', ( #6589, #3130, #5413, #7186 ) ) ;
#3647=ORIENTED_EDGE ( 'NONE', *, *, #542, .T. ) ;
#3649=CARTESIAN_POINT ( 'NONE',  ( 38.19229777560031636, 37.08684478514405214, 12.50000000000000000 ) ) ;
#3651=DIRECTION ( 'NONE',  ( 0.000000000000000000, 0.000000000000000000, 1.000000000000000000 ) ) ;
#3656=EDGE_CURVE ( 'NONE', #2894, #426, #5349, .T. ) ;
#3657=ORIENTED_EDGE ( 'NONE', *, *, #6508, .T. ) ;
#3658=EDGE_CURVE ( 'NONE', #8983, #3675, #5363, .T. ) ;
#3661=AXIS2_PLACEMENT_3D ( 'NONE', #9077, #8336, #135 ) ;
#3665=FACE_OUTER_BOUND ( 'NONE', #3217, .T. ) ;
#3670=EDGE_CURVE ( 'NONE', #2404, #5066, #3579, .T. ) ;
#3672=AXIS2_PLACEMENT_3D ( 'NONE', #8927, #8180, #8075 ) ;
#3675=VERTEX_POINT ( 'NONE', #4689 ) ;
#3676=DIRECTION ( 'NONE',  ( -0.000000000000000000, -0.000000000000000000, -1.000000000000000000 ) ) ;
#3677=LINE ( 'NONE', #6795, #9681 ) ;
#3679=CARTESIAN_POINT ( 'NONE',  ( -27.15769640663939555, -115.1457019118818863, -27.15769640663944173 ) ) ;
#3681=AXIS2_PLACEMENT_3D ( 'NONE', #227, #8432, #6191 ) ;
#3684=ORIENTED_EDGE ( 'NONE', *, *, #2170, .T. ) ;
#3685=LINE ( 'NONE', #3469, #9543 ) ;
#3687=CARTESIAN_POINT ( 'NONE',  ( 0.000000000000000000, -145.1457019118819005, -50.00000000000002132 ) ) ;
#3691=AXIS2_PLACEMENT_3D ( 'NONE', #2240, #8647, #4723 ) ;
#3692=DIRECTION ( 'NONE',  ( -0.000000000000000000, 1.000000000000000000, -0.000000000000000000 ) ) ;
#3699=VERTEX_POINT ( 'NONE', #1297 ) ;
#3701=ORIENTED_EDGE ( 'NONE', *, *, #8365, .T. ) ;
#3703=CYLINDRICAL_SURFACE ( 'NONE', #3836, 4.999999999999996447 ) ;
#3704=DIRECTION ( 'NONE',  ( 0.000000000000000000, 0.000000000000000000, 1.000000000000000000 ) ) ;
#3705=EDGE_LOOP ( 'NONE', ( #5798, #10329, #6997, #7020 ) ) ;
#3710=VERTEX_POINT ( 'NONE', #5319 ) ;
#3711=VECTOR ( 'NONE', #1031, 1000.000000000000000 ) ;
#3714=ORIENTED_EDGE ( 'NONE', *, *, #9165, .F. ) ;
#3717=CIRCLE ( 'NONE', #1178, 2.000000000000001776 ) ;
#3718=DIRECTION ( 'NONE',  ( -1.000000000000000000, -0.000000000000000000, -0.000000000000000000 ) ) ;
#3722=ORIENTED_EDGE ( 'NONE', *, *, #5846, .F. ) ;
#3724=CIRCLE ( 'NONE', #3855, 4.000000000000000000 ) ;
#3725=ORIENTED_EDGE ( 'NONE', *, *, #1009, .F. ) ;
#3732=ADVANCED_FACE ( 'NONE', ( #8771 ), #8716, .F. ) ;
#3736=CARTESIAN_POINT ( 'NONE',  ( 59.99999999999999289, -145.1457019118819005, -40.00000000000000000 ) ) ;
#3737=DIRECTION ( 'NONE',  ( -1.000000000000000000, 0.000000000000000000, 1.396588258780021135E-16 ) ) ;
#3740=FACE_OUTER_BOUND ( 'NONE', #3994, .T. ) ;
#3742=VERTEX_POINT ( 'NONE', #5479 ) ;
#3749=VERTEX_POINT ( 'NONE', #8661 ) ;
#3751=LINE ( 'NONE', #9536, #5778 ) ;
#3754=CARTESIAN_POINT ( 'NONE',  ( 23.76520584195949226, -145.1457019118819005, -97.78965767959371647 ) ) ;
#3755=DIRECTION ( 'NONE',  ( 0.000000000000000000, 0.000000000000000000, -1.000000000000000000 ) ) ;
#3756=CARTESIAN_POINT ( 'NONE',  ( -27.15769640663937778, -133.1457019118818721, -48.00000000000002132 ) ) ;
#3757=CARTESIAN_POINT ( 'NONE',  ( -23.15769640663940976, -115.1457019118818863, 47.99999999999997868 ) ) ;
#3759=VECTOR ( 'NONE', #2544, 1000.000000000000000 ) ;
#3765=CARTESIAN_POINT ( 'NONE',  ( -16.29350689640809691, -140.1746510883711778, 30.31717237747080773 ) ) ;
#3766=CARTESIAN_POINT ( 'NONE',  ( 23.15769640663940265, -133.1457019118818721, -48.00000000000002132 ) ) ;
#3769=CARTESIAN_POINT ( 'NONE',  ( 17.97972049165455388, 17.84145331825995484, -12.49999999999999289 ) ) ;
#3773=ORIENTED_EDGE ( 'NONE', *, *, #457, .F. ) ;
#3775=AXIS2_PLACEMENT_3D ( 'NONE', #7809, #5579, #1451 ) ;
#3776=EDGE_CURVE ( 'NONE', #6574, #9783, #6167, .T. ) ;
#3778=EDGE_LOOP ( 'NONE', ( #766, #6098, #5752, #7906 ) ) ;
#3781=LINE ( 'NONE', #3568, #1631 ) ;
#3783=AXIS2_PLACEMENT_3D ( 'NONE', #4610, #8799, #4663 ) ;
#3785=VERTEX_POINT ( 'NONE', #9357 ) ;
#3786=DIRECTION ( 'NONE',  ( 1.000000000000000000, 0.000000000000000000, 8.379529552680125332E-16 ) ) ;
#3788=EDGE_CURVE ( 'NONE', #7130, #3710, #9961, .T. ) ;
#3791=DIRECTION ( 'NONE',  ( 8.379529552680125332E-16, 0.000000000000000000, -1.000000000000000000 ) ) ;
#3792=ORIENTED_EDGE ( 'NONE', *, *, #10398, .T. ) ;
#3794=CYLINDRICAL_SURFACE ( 'NONE', #1933, 3.297986701801175258 ) ;
#3795=CARTESIAN_POINT ( 'NONE',  ( -40.00000000000002842, -145.1457019118819005, 43.99999999999997158 ) ) ;
#3801=ORIENTED_EDGE ( 'NONE', *, *, #6715, .F. ) ;
#3803=DIRECTION ( 'NONE',  ( 0.000000000000000000, 0.000000000000000000, 1.000000000000000000 ) ) ;
#3808=DIRECTION ( 'NONE',  ( -1.000000000000000000, 0.000000000000000000, 0.000000000000000000 ) ) ;
#3810=CARTESIAN_POINT ( 'NONE',  ( 27.15769640663936713, -115.1457019118818863, 27.15769640663938489 ) ) ;
#3812=DIRECTION ( 'NONE',  ( -1.000000000000000000, 0.000000000000000000, -1.396588258780018177E-16 ) ) ;
#3813=FACE_OUTER_BOUND ( 'NONE', #9404, .T. ) ;
#3815=CIRCLE ( 'NONE', #5156, 3.297986701801175258 ) ;
#3819=ORIENTED_EDGE ( 'NONE', *, *, #9237, .T. ) ;
#3820=DIRECTION ( 'NONE',  ( -1.000000000000000000, 0.000000000000000000, 0.000000000000000000 ) ) ;
#3829=AXIS2_PLACEMENT_3D ( 'NONE', #3425, #4065, #9853 ) ;
#3831=EDGE_LOOP ( 'NONE', ( #743, #377, #7548, #3998, #6128, #388, #8707, #110, #8384, #2626 ) ) ;
#3836=AXIS2_PLACEMENT_3D ( 'NONE', #8466, #4336, #8415 ) ;
#3837=EDGE_CURVE ( 'NONE', #8, #4758, #957, .T. ) ;
#3838=CARTESIAN_POINT ( 'NONE',  ( -48.00000000000002132, -135.1457019118818721, 23.15769640663938134 ) ) ;
#3839=AXIS2_PLACEMENT_3D ( 'NONE', #6429, #762, #7445 ) ;
#3840=VERTEX_POINT ( 'NONE', #4295 ) ;
#3843=VERTEX_POINT ( 'NONE', #1753 ) ;
#3848=CARTESIAN_POINT ( 'NONE',  ( 73.53765631853929108, 70.39106037767955115, -25.00000000000000355 ) ) ;
#3849=EDGE_CURVE ( 'NONE', #7537, #4871, #1700, .T. ) ;
#3850=DIRECTION ( 'NONE',  ( -1.000000000000000000, 0.000000000000000000, 0.000000000000000000 ) ) ;
#3853=ORIENTED_EDGE ( 'NONE', *, *, #5767, .F. ) ;
#3854=DIRECTION ( 'NONE',  ( 1.000000000000000000, 0.000000000000000000, -1.396588258780018177E-16 ) ) ;
#3855=AXIS2_PLACEMENT_3D ( 'NONE', #2160, #7196, #3864 ) ;
#3859=ORIENTED_EDGE ( 'NONE', *, *, #6309, .T. ) ;
#3860=TOROIDAL_SURFACE ( 'NONE', #8590, 4.000000000000000000, 2.000000000000000000 ) ;
#3863=CARTESIAN_POINT ( 'NONE',  ( 39.99999999999997158, -135.1457019118818721, 35.97499999999998010 ) ) ;
#3864=DIRECTION ( 'NONE',  ( 0.000000000000000000, 0.000000000000000000, 1.000000000000000000 ) ) ;
#3865=CIRCLE ( 'NONE', #3171, 4.000000000000000000 ) ;
#3869=DIRECTION ( 'NONE',  ( 0.000000000000000000, 0.000000000000000000, -1.000000000000000000 ) ) ;
#3871=CARTESIAN_POINT ( 'NONE',  ( -2.293506896408097795, 152.5696653505793279, 30.00000000000000355 ) ) ;
#3878=CARTESIAN_POINT ( 'NONE',  ( -48.00000000000002132, -117.1457019118819005, 23.15769640663938134 ) ) ;
#3879=DIRECTION ( 'NONE',  ( 0.000000000000000000, 0.000000000000000000, 1.000000000000000000 ) ) ;
#3880=CIRCLE ( 'NONE', #4870, 7.500000000000000000 ) ;
#3881=ORIENTED_EDGE ( 'NONE', *, *, #1213, .F. ) ;
#3882=LINE ( 'NONE', #3974, #1912 ) ;
#3883=CYLINDRICAL_SURFACE ( 'NONE', #7851, 4.000000000000000000 ) ;
#3887=ORIENTED_EDGE ( 'NONE', *, *, #995, .F. ) ;
#3888=ADVANCED_FACE ( 'NONE', ( #8377 ), #6902, .F. ) ;
#3889=ORIENTED_EDGE ( 'NONE', *, *, #2696, .T. ) ;
#3893=CARTESIAN_POINT ( 'NONE',  ( 24.15108826162069633, -134.0910007290636941, 49.99999999999998579 ) ) ;
#3897=ORIENTED_EDGE ( 'NONE', *, *, #3656, .F. ) ;
#3901=ORIENTED_EDGE ( 'NONE', *, *, #5304, .T. ) ;
#3904=LINE ( 'NONE', #9580, #424 ) ;
#3905=LINE ( 'NONE', #1410, #7547 ) ;
#3906=ORIENTED_EDGE ( 'NONE', *, *, #7396, .T. ) ;
#3910=CARTESIAN_POINT ( 'NONE',  ( -18.34874108452141783, -140.1746510883711778, -97.78965767959371647 ) ) ;
#3913=ORIENTED_EDGE ( 'NONE', *, *, #9379, .F. ) ;
#3921=ORIENTED_EDGE ( 'NONE', *, *, #6509, .T. ) ;
#3922=DIRECTION ( 'NONE',  ( 0.000000000000000000, 0.000000000000000000, -1.000000000000000000 ) ) ;
#3923=AXIS2_PLACEMENT_3D ( 'NONE', #7508, #3426, #256 ) ;
#3926=EDGE_CURVE ( 'NONE', #3983, #9491, #2830, .T. ) ;
#3928=DIRECTION ( 'NONE',  ( 3.469446951953611033E-15, -1.000000000000000000, 0.000000000000000000 ) ) ;
#3931=FACE_OUTER_BOUND ( 'NONE', #1363, .T. ) ;
#3934=EDGE_LOOP ( 'NONE', ( #7042, #7343, #4080, #1301 ) ) ;
#3935=AXIS2_PLACEMENT_3D ( 'NONE', #10224, #8073, #1609 ) ;
#3936=ORIENTED_EDGE ( 'NONE', *, *, #2427, .T. ) ;
#3937=EDGE_CURVE ( 'NONE', #3587, #4776, #9622, .T. ) ;
#3938=AXIS2_PLACEMENT_3D ( 'NONE', #3186, #7170, #10454 ) ;
#3939=DIRECTION ( 'NONE',  ( 1.000000000000000000, 1.277197683604454965E-16, -0.000000000000000000 ) ) ;
#3943=CARTESIAN_POINT ( 'NONE',  ( 17.97972049165455388, 17.84145331825995484, 12.50000000000000355 ) ) ;
#3946=AXIS2_PLACEMENT_3D ( 'NONE', #6228, #2147, #3854 ) ;
#3949=DIRECTION ( 'NONE',  ( 0.000000000000000000, -1.000000000000000000, 0.000000000000000000 ) ) ;
#3952=CARTESIAN_POINT ( 'NONE',  ( 38.19229777560031636, 37.08684478514405214, -12.50000000000000000 ) ) ;
#3956=CYLINDRICAL_SURFACE ( 'NONE', #3946, 2.000000000000001776 ) ;
#3957=VECTOR ( 'NONE', #7464, 1000.000000000000000 ) ;
#3964=CARTESIAN_POINT ( 'NONE',  ( -16.29350689640809691, -186.9457019118818835, -7.500000000000000000 ) ) ;
#3965=PLANE ( 'NONE',  #3135 ) ;
#3968=EDGE_CURVE ( 'NONE', #7191, #7421, #3865, .T. ) ;
#3969=ORIENTED_EDGE ( 'NONE', *, *, #1213, .T. ) ;
#3971=DIRECTION ( 'NONE',  ( -0.000000000000000000, 1.000000000000000000, -0.000000000000000000 ) ) ;
#3974=CARTESIAN_POINT ( 'NONE',  ( -50.00000000000002842, -117.1457019118819005, 25.15769640663938134 ) ) ;
#3976=AXIS2_PLACEMENT_3D ( 'NONE', #2355, #81, #137 ) ;
#3978=ORIENTED_EDGE ( 'NONE', *, *, #3367, .T. ) ;
#3983=VERTEX_POINT ( 'NONE', #9444 ) ;
#3987=CARTESIAN_POINT ( 'NONE',  ( -18.34874108452141783, -140.1746510883711778, -29.59847408863698703 ) ) ;
#3990=ADVANCED_FACE ( 'NONE', ( #8480 ), #4350, .T. ) ;
#3993=EDGE_CURVE ( 'NONE', #6699, #2463, #381, .T. ) ;
#3994=EDGE_LOOP ( 'NONE', ( #1326, #5964, #298, #8127 ) ) ;
#3995=AXIS2_PLACEMENT_3D ( 'NONE', #2578, #5805, #829 ) ;
#3998=ORIENTED_EDGE ( 'NONE', *, *, #655, .T. ) ;
#4003=CARTESIAN_POINT ( 'NONE',  ( 37.36731276015125758, -134.9005680707593342, -26.18936614083822434 ) ) ;
#4004=EDGE_CURVE ( 'NONE', #5912, #5230, #533, .T. ) ;
#4005=ORIENTED_EDGE ( 'NONE', *, *, #3402, .F. ) ;
#4006=FACE_OUTER_BOUND ( 'NONE', #865, .T. ) ;
#4013=ORIENTED_EDGE ( 'NONE', *, *, #10070, .F. ) ;
#4014=VECTOR ( 'NONE', #4958, 1000.000000000000000 ) ;
#4015=CARTESIAN_POINT ( 'NONE',  ( -16.29350689640809691, -115.1457019118818863, 0.000000000000000000 ) ) ;
#4016=CARTESIAN_POINT ( 'NONE',  ( 14.70649310359190309, 120.5696653505793705, -24.00000000000000711 ) ) ;
#4017=DIRECTION ( 'NONE',  ( -8.379529552680125332E-16, 0.000000000000000000, 1.000000000000000000 ) ) ;
#4019=AXIS2_PLACEMENT_3D ( 'NONE', #5221, #352, #2678 ) ;
#4022=AXIS2_PLACEMENT_3D ( 'NONE', #760, #8814, #7131 ) ;
#4023=LINE ( 'NONE', #7254, #4351 ) ;
#4026=LINE ( 'NONE', #2477, #4209 ) ;
#4028=CARTESIAN_POINT ( 'NONE',  ( -23.15769640663940621, -115.1457019118818863, 27.15769640663938489 ) ) ;
#4029=DIRECTION ( 'NONE',  ( 0.000000000000000000, 1.000000000000000000, 0.000000000000000000 ) ) ;
#4030=CARTESIAN_POINT ( 'NONE',  ( 27.15769640663936713, -133.1457019118818721, 27.15769640663938489 ) ) ;
#4032=ORIENTED_EDGE ( 'NONE', *, *, #5381, .T. ) ;
#4033=AXIS2_PLACEMENT_3D ( 'NONE', #8272, #5719, #116 ) ;
#4034=ORIENTED_EDGE ( 'NONE', *, *, #5304, .F. ) ;
#4035=EDGE_CURVE ( 'NONE', #6316, #2974, #650, .T. ) ;
#4036=CARTESIAN_POINT ( 'NONE',  ( -50.00000000000002132, -134.0910177696405015, -24.15110854952568431 ) ) ;
#4037=EDGE_CURVE ( 'NONE', #3587, #836, #3613, .T. ) ;
#4039=CIRCLE ( 'NONE', #8094, 4.025000000000000355 ) ;
#4041=ORIENTED_EDGE ( 'NONE', *, *, #8365, .F. ) ;
#4043=ORIENTED_EDGE ( 'NONE', *, *, #7223, .F. ) ;
#4044=DIRECTION ( 'NONE',  ( 1.000000000000000000, -0.000000000000000000, -0.000000000000000000 ) ) ;
#4045=AXIS2_PLACEMENT_3D ( 'NONE', #9883, #9070, #2501 ) ;
#4046=VERTEX_POINT ( 'NONE', #9335 ) ;
#4047=VERTEX_POINT ( 'NONE', #6040 ) ;
#4050=EDGE_CURVE ( 'NONE', #1239, #7344, #4529, .T. ) ;
#4052=CARTESIAN_POINT ( 'NONE',  ( 17.97972049165455388, 42.08684478514406635, 30.00000000000000355 ) ) ;
#4053=VECTOR ( 'NONE', #3223, 1000.000000000000000 ) ;
#4055=CARTESIAN_POINT ( 'NONE',  ( 37.24181578876673626, -134.1736247882644193, -25.42151319394753628 ) ) ;
#4065=DIRECTION ( 'NONE',  ( 0.000000000000000000, -1.000000000000000000, 0.000000000000000000 ) ) ;
#4066=FACE_OUTER_BOUND ( 'NONE', #7268, .T. ) ;
#4067=DIRECTION ( 'NONE',  ( -1.277197683604454965E-16, 1.000000000000000000, -0.000000000000000000 ) ) ;
#4068=EDGE_LOOP ( 'NONE', ( #3881, #528, #844, #8698 ) ) ;
#4073=LINE ( 'NONE', #8896, #1073 ) ;
#4075=CARTESIAN_POINT ( 'NONE',  ( -16.29350689640809691, -140.1746510883711778, -23.72119897386845722 ) ) ;
#4076=VERTEX_POINT ( 'NONE', #2120 ) ;
#4080=ORIENTED_EDGE ( 'NONE', *, *, #7480, .F. ) ;
#4082=CARTESIAN_POINT ( 'NONE',  ( 27.15769640663937068, -135.1457019118818721, 47.99999999999997868 ) ) ;
#4083=DIRECTION ( 'NONE',  ( 0.000000000000000000, -1.000000000000000000, 0.000000000000000000 ) ) ;
#4084=VECTOR ( 'NONE', #3254, 1000.000000000000000 ) ;
#4089=VERTEX_POINT ( 'NONE', #2016 ) ;
#4091=ORIENTED_EDGE ( 'NONE', *, *, #7423, .F. ) ;
#4092=DIRECTION ( 'NONE',  ( -0.000000000000000000, -0.000000000000000000, 1.000000000000000000 ) ) ;
#4100=DIRECTION ( 'NONE',  ( -1.277197683604454965E-16, 1.000000000000000000, 0.000000000000000000 ) ) ;
#4101=AXIS2_PLACEMENT_3D ( 'NONE', #10014, #5176, #9265 ) ;
#4102=VECTOR ( 'NONE', #3537, 1000.000000000000000 ) ;
#4103=CARTESIAN_POINT ( 'NONE',  ( 37.59878849545336976, 32.08684478514406635, 12.50000000000000355 ) ) ;
#4116=DIRECTION ( 'NONE',  ( 8.659560562356134638E-17, 0.7071067811864494290, -0.7071067811866454944 ) ) ;
#4118=VECTOR ( 'NONE', #5192, 1000.000000000000000 ) ;
#4120=CARTESIAN_POINT ( 'NONE',  ( 59.99999999999997868, -135.1457019118818721, 30.00000000000000355 ) ) ;
#4122=ADVANCED_FACE ( 'NONE', ( #2284 ), #1826, .F. ) ;
#4125=AXIS2_PLACEMENT_3D ( 'NONE', #6081, #521, #1104 ) ;
#4128=CARTESIAN_POINT ( 'NONE',  ( 17.97972049165455388, 37.08684478514406635, -24.99999999999998934 ) ) ;
#4129=DIRECTION ( 'NONE',  ( 0.000000000000000000, 0.000000000000000000, -1.000000000000000000 ) ) ;
#4131=CARTESIAN_POINT ( 'NONE',  ( 49.99999999999998579, -135.1457019118818721, -40.00000000000002132 ) ) ;
#4134=CIRCLE ( 'NONE', #6665, 4.000000000000000000 ) ;
#4139=ADVANCED_FACE ( 'NONE', ( #6257 ), #790, .F. ) ;
#4140=CIRCLE ( 'NONE', #1267, 3.999999999999996447 ) ;
#4145=ORIENTED_EDGE ( 'NONE', *, *, #8155, .T. ) ;
#4148=ORIENTED_EDGE ( 'NONE', *, *, #3611, .F. ) ;
#4151=LINE ( 'NONE', #3515, #3236 ) ;
#4154=EDGE_CURVE ( 'NONE', #5439, #8294, #4814, .T. ) ;
#4159=DIRECTION ( 'NONE',  ( 0.000000000000000000, -0.000000000000000000, 1.000000000000000000 ) ) ;
#4162=CARTESIAN_POINT ( 'NONE',  ( 0.000000000000000000, -117.1457019118819005, -48.00000000000002132 ) ) ;
#4163=ORIENTED_EDGE ( 'NONE', *, *, #1275, .F. ) ;
#4168=VECTOR ( 'NONE', #6267, 1000.000000000000000 ) ;
#4169=DIRECTION ( 'NONE',  ( 0.000000000000000000, 0.000000000000000000, -1.000000000000000000 ) ) ;
#4170=CARTESIAN_POINT ( 'NONE',  ( 94.78677303995212355, -145.1457019118819005, -30.00000000000000355 ) ) ;
#4173=LINE ( 'NONE', #7408, #4685 ) ;
#4174=AXIS2_PLACEMENT_3D ( 'NONE', #4905, #9654, #835 ) ;
#4175=ORIENTED_EDGE ( 'NONE', *, *, #7223, .T. ) ;
#4180=AXIS2_PLACEMENT_3D ( 'NONE', #9670, #123, #3356 ) ;
#4181=ADVANCED_FACE ( 'NONE', ( #7059 ), #693, .F. ) ;
#4183=CARTESIAN_POINT ( 'NONE',  ( -16.29350689640809691, -115.1457019118818863, 7.500000000000000000 ) ) ;
#4184=CARTESIAN_POINT ( 'NONE',  ( 1.940506014114294486E-14, -117.1457019118819005, -23.15769640663942752 ) ) ;
#4190=ORIENTED_EDGE ( 'NONE', *, *, #7208, .F. ) ;
#4192=LINE ( 'NONE', #1807, #9868 ) ;
#4193=VECTOR ( 'NONE', #9291, 1000.000000000000000 ) ;
#4194=EDGE_CURVE ( 'NONE', #5490, #4722, #7874, .T. ) ;
#4196=CARTESIAN_POINT ( 'NONE',  ( -2.293506896408097795, 80.56966535057935630, 20.00000000000000711 ) ) ;
#4204=UNCERTAINTY_MEASURE_WITH_UNIT (LENGTH_MEASURE( 1.000000000000000082E-05 ), #520, 'distance_accuracy_value', 'NONE');
#4205=DIRECTION ( 'NONE',  ( 0.000000000000000000, 0.000000000000000000, -1.000000000000000000 ) ) ;
#4207=DIRECTION ( 'NONE',  ( 0.000000000000000000, 0.000000000000000000, 1.000000000000000000 ) ) ;
#4208=LINE ( 'NONE', #2617, #8167 ) ;
#4209=VECTOR ( 'NONE', #6453, 1000.000000000000000 ) ;
#4211=DIRECTION ( 'NONE',  ( -0.000000000000000000, 1.000000000000000000, -0.000000000000000000 ) ) ;
#4214=DIRECTION ( 'NONE',  ( -0.000000000000000000, -0.000000000000000000, 1.000000000000000000 ) ) ;
#4215=EDGE_CURVE ( 'NONE', #6531, #10235, #6488, .T. ) ;
#4217=ORIENTED_EDGE ( 'NONE', *, *, #1064, .T. ) ;
#4221=CARTESIAN_POINT ( 'NONE',  ( 27.15769640663936713, -135.1457019118818721, 27.15769640663938489 ) ) ;
#4222=CARTESIAN_POINT ( 'NONE',  ( -40.00000000000002842, -135.1457019118818721, 35.97499999999998010 ) ) ;
#4223=CYLINDRICAL_SURFACE ( 'NONE', #5329, 4.000000000000000000 ) ;
#4227=ADVANCED_FACE ( 'NONE', ( #644 ), #3883, .F. ) ;
#4230=ORIENTED_EDGE ( 'NONE', *, *, #2184, .T. ) ;
#4235=DIRECTION ( 'NONE',  ( -1.000000000000000000, 0.000000000000000000, 0.000000000000000000 ) ) ;
#4238=EDGE_CURVE ( 'NONE', #5439, #5589, #9609, .T. ) ;
#4245=VECTOR ( 'NONE', #4598, 1000.000000000000000 ) ;
#4248=EDGE_LOOP ( 'NONE', ( #8890, #7075, #4673, #6353 ) ) ;
#4251=EDGE_LOOP ( 'NONE', ( #5455, #515, #8987 ) ) ;
#4253=ORIENTED_EDGE ( 'NONE', *, *, #8525, .T. ) ;
#4256=DIRECTION ( 'NONE',  ( -1.000000000000000000, 0.000000000000000000, 0.000000000000000000 ) ) ;
#4257=CARTESIAN_POINT ( 'NONE',  ( -2.293506896408097795, 120.5696653505793705, 24.00000000000000711 ) ) ;
#4259=CARTESIAN_POINT ( 'NONE',  ( -23.76520584195948516, -145.1457019118819005, 0.6509338422959615178 ) ) ;
#4262=CIRCLE ( 'NONE', #1727, 4.999999999999997335 ) ;
#4263=DIRECTION ( 'NONE',  ( -1.396588258780021135E-16, 0.000000000000000000, -1.000000000000000000 ) ) ;
#4264=EDGE_LOOP ( 'NONE', ( #913, #7746, #6785, #9673, #8190, #8904, #1504, #8985 ) ) ;
#4265=DIRECTION ( 'NONE',  ( 0.000000000000000000, -1.000000000000000000, 0.000000000000000000 ) ) ;
#4268=( BOUNDED_CURVE ( )  B_SPLINE_CURVE ( 3, ( #6344, #7828, #6130, #8674 ),
 .UNSPECIFIED., .F., .T. ) 
 B_SPLINE_CURVE_WITH_KNOTS ( ( 4, 4 ),
 ( 2.243596561310086113, 4.039588745869489017 ),
 .UNSPECIFIED. ) 
 CURVE ( )  GEOMETRIC_REPRESENTATION_ITEM ( )  RATIONAL_B_SPLINE_CURVE ( ( 1.000000000000000000, 0.7487856226529292503, 0.7487856226529292503, 1.000000000000000000 ) ) 
 REPRESENTATION_ITEM ( '' )  );
#4270=CARTESIAN_POINT ( 'NONE',  ( 94.78677303995212355, -145.1457019118819005, 30.00000000000000355 ) ) ;
#4271=CARTESIAN_POINT ( 'NONE',  ( 14.70649310359190309, 80.56966535057935630, 20.00000000000000711 ) ) ;
#4273=CARTESIAN_POINT ( 'NONE',  ( 27.15769640663938489, -117.1457019118819005, -27.15769640663940976 ) ) ;
#4275=AXIS2_PLACEMENT_3D ( 'NONE', #8441, #547, #8550 ) ;
#4279=CARTESIAN_POINT ( 'NONE',  ( -16.29350689640809691, -115.1457019118818863, -7.500000000000000000 ) ) ;
#4280=EDGE_LOOP ( 'NONE', ( #7317, #130, #4013, #9753 ) ) ;
#4283=DIRECTION ( 'NONE',  ( 0.000000000000000000, 0.000000000000000000, 1.000000000000000000 ) ) ;
#4285=EDGE_CURVE ( 'NONE', #9459, #3359, #3339, .T. ) ;
#4286=DIRECTION ( 'NONE',  ( -0.000000000000000000, -0.000000000000000000, -1.000000000000000000 ) ) ;
#4290=ORIENTED_EDGE ( 'NONE', *, *, #9363, .T. ) ;
#4295=CARTESIAN_POINT ( 'NONE',  ( 39.99999999999998579, -145.1457019118819005, -44.00000000000001421 ) ) ;
#4297=ADVANCED_FACE ( 'NONE', ( #6671 ), #6567, .T. ) ;
#4301=ORIENTED_EDGE ( 'NONE', *, *, #817, .F. ) ;
#4303=AXIS2_PLACEMENT_3D ( 'NONE', #10260, #1355, #2938 ) ;
#4305=CARTESIAN_POINT ( 'NONE',  ( 6.756858349438843447, 146.7073643690756057, 30.00000000000000355 ) ) ;
#4306=DIRECTION ( 'NONE',  ( -0.000000000000000000, 1.000000000000000000, -0.000000000000000000 ) ) ;
#4307=CARTESIAN_POINT ( 'NONE',  ( 27.15769640663938489, -115.1457019118818863, -23.15769640663940976 ) ) ;
#4311=EDGE_CURVE ( 'NONE', #172, #541, #5323, .T. ) ;
#4313=DIRECTION ( 'NONE',  ( -0.7367503238654704578, 0.6761648913424330720, 0.000000000000000000 ) ) ;
#4318=VERTEX_POINT ( 'NONE', #9813 ) ;
#4323=ADVANCED_FACE ( 'NONE', ( #8310 ), #1048, .T. ) ;
#4324=DIRECTION ( 'NONE',  ( 0.000000000000000000, 0.000000000000000000, 1.000000000000000000 ) ) ;
#4325=DIRECTION ( 'NONE',  ( 0.000000000000000000, 0.000000000000000000, 1.000000000000000000 ) ) ;
#4331=EDGE_CURVE ( 'NONE', #3508, #3054, #9914, .T. ) ;
#4332=EDGE_LOOP ( 'NONE', ( #8016, #10231, #6035, #2761 ) ) ;
#4336=DIRECTION ( 'NONE',  ( -0.07334937666141726209, 0.9973063064792991872, 0.000000000000000000 ) ) ;
#4337=CARTESIAN_POINT ( 'NONE',  ( 27.15769640663938489, -133.1457019118818721, -27.15769640663940976 ) ) ;
#4339=DIRECTION ( 'NONE',  ( -1.000000000000000000, 0.000000000000000000, 0.000000000000000000 ) ) ;
#4341=VECTOR ( 'NONE', #4573, 1000.000000000000000 ) ;
#4345=VECTOR ( 'NONE', #1374, 1000.000000000000000 ) ;
#4346=CIRCLE ( 'NONE', #10443, 7.500000000000000000 ) ;
#4349=CARTESIAN_POINT ( 'NONE',  ( -50.00000000000001421, -133.3869996355352612, 23.39899473323094270 ) ) ;
#4350=PLANE ( 'NONE',  #312 ) ;
#4351=VECTOR ( 'NONE', #3219, 1000.000000000000000 ) ;
#4353=LINE ( 'NONE', #9932, #5011 ) ;
#4355=CIRCLE ( 'NONE', #5021, 7.500000000000000000 ) ;
#4359=CLOSED_SHELL ( 'NONE', ( #570, #7878, #6208, #9860, #857, #7865, #4139, #616, #2359, #1611, #10351, #4888, #4743, #9567, #3888, #8424, #8714, #8844, #4684, #6762, #1759, #3606, #529, #1901, #4563, #6970, #180, #30, #5472, #2811, #4846, #9628, #3331, #4323, #3732, #3553, #5399, #9690, #6969, #6687, #7252, #3346, #3990, #5024, #3539, #10015, #8672, #580, #5441, #2738, #5395, #9483, #6108, #1261, #1338, #1569, #9965, #8065, #3399, #5238, #7805, #1995, #4122, #5525, #5081, #6380, #9752, #8493, #10341, #1806, #2351, #5754, #1350, #8888, #8902, #7762, #9828, #10452, #1657, #6411, #6946, #5157, #4992, #4181, #9352, #7221, #2361, #6026, #4227, #870, #3051, #5237, #4695, #5652, #8727, #10467, #936, #4389, #9803, #2045, #8816, #9290, #1582, #2753, #7232, #1726, #9243, #6109, #3080, #1335, #4966, #1470, #949, #9627, #9407, #4297, #9231, #5699, #6899, #10025, #7852, #3195, #9599, #9039, #7287, #6836, #921, #6171, #8037, #6187, #223, #2825, #3463, #196, #64, #6263, #3432, #9766, #9081, #10261, #8391, #2880, #1396, #4562, #4574, #7482, #8906, #6392 ) ) ;
#4360=VERTEX_POINT ( 'NONE', #5709 ) ;
#4365=DIRECTION ( 'NONE',  ( 1.000000000000000000, 0.000000000000000000, 0.000000000000000000 ) ) ;
#4367=CARTESIAN_POINT ( 'NONE',  ( 77.30044127146538813, 73.68369600860394542, 12.50000000000000000 ) ) ;
#4374=EDGE_CURVE ( 'NONE', #59, #7038, #8100, .T. ) ;
#4375=EDGE_CURVE ( 'NONE', #1149, #2894, #1797, .T. ) ;
#4378=VECTOR ( 'NONE', #1273, 1000.000000000000000 ) ;
#4379=LINE ( 'NONE', #8348, #9954 ) ;
#4382=LINE ( 'NONE', #5266, #7709 ) ;
#4384=ORIENTED_EDGE ( 'NONE', *, *, #2895, .F. ) ;
#4386=VERTEX_POINT ( 'NONE', #4131 ) ;
#4388=ORIENTED_EDGE ( 'NONE', *, *, #7256, .F. ) ;
#4389=ADVANCED_FACE ( 'NONE', ( #8209 ), #6616, .T. ) ;
#4393=CARTESIAN_POINT ( 'NONE',  ( -48.00000000000002132, -115.1457019118818863, -6.661338147750942398E-15 ) ) ;
#4395=B_SPLINE_CURVE_WITH_KNOTS ( 'NONE', 3,
 ( #9087, #8242, #5000, #7395, #4896, #7342, #8986, #1673, #2572, #872 ),
 .UNSPECIFIED., .F., .F.,
 ( 4, 2, 2, 2, 4 ),
 ( -8.944271910636758738E-06, 0.001019331502940711920, 0.002047607277792060521, 0.003075883052643409339, 0.004104158827494757723 ),
 .UNSPECIFIED. ) ;
#4398=CARTESIAN_POINT ( 'NONE',  ( -2.293506896408097795, 80.56966535057935630, -24.00000000000000711 ) ) ;
#4400=VERTEX_POINT ( 'NONE', #1001 ) ;
#4403=CARTESIAN_POINT ( 'NONE',  ( 0.000000000000000000, -117.1457019118819005, 23.15769640663938134 ) ) ;
#4404=CARTESIAN_POINT ( 'NONE',  ( -50.00000000000002132, -133.1457019118818721, 23.15769640663938134 ) ) ;
#4407=VERTEX_POINT ( 'NONE', #5922 ) ;
#4408=CARTESIAN_POINT ( 'NONE',  ( 4.856471286862175774, 147.5696653505793279, 30.00000000000000355 ) ) ;
#4415=DIRECTION ( 'NONE',  ( 0.000000000000000000, 0.000000000000000000, 1.000000000000000000 ) ) ;
#4416=EDGE_LOOP ( 'NONE', ( #6142, #3010, #4145, #1095, #10153, #9819, #3055, #6388, #3078, #9041, #7776, #5214 ) ) ;
#4419=VERTEX_POINT ( 'NONE', #8470 ) ;
#4421=EDGE_LOOP ( 'NONE', ( #6149, #8118, #539, #375 ) ) ;
#4422=VECTOR ( 'NONE', #4860, 1000.000000000000114 ) ;
#4430=EDGE_LOOP ( 'NONE', ( #9412, #7534, #9123, #2319 ) ) ;
#4431=DIRECTION ( 'NONE',  ( -0.000000000000000000, -0.000000000000000000, -1.000000000000000000 ) ) ;
#4432=VERTEX_POINT ( 'NONE', #10019 ) ;
#4433=ORIENTED_EDGE ( 'NONE', *, *, #4646, .F. ) ;
#4434=AXIS2_PLACEMENT_3D ( 'NONE', #2692, #7571, #321 ) ;
#4436=VECTOR ( 'NONE', #1392, 1000.000000000000000 ) ;
#4437=VERTEX_POINT ( 'NONE', #10173 ) ;
#4438=CARTESIAN_POINT ( 'NONE',  ( -40.00000000000002842, -115.1457019118818863, 39.99999999999997868 ) ) ;
#4440=ORIENTED_EDGE ( 'NONE', *, *, #8077, .T. ) ;
#4445=CARTESIAN_POINT ( 'NONE',  ( 80.08610854271792334, 54.73418909528891874, -25.00000000000000355 ) ) ;
#4448=LINE ( 'NONE', #4497, #4746 ) ;
#4451=ORIENTED_EDGE ( 'NONE', *, *, #6760, .T. ) ;
#4454=ORIENTED_EDGE ( 'NONE', *, *, #3096, .F. ) ;
#4458=DIRECTION ( 'NONE',  ( -1.000000000000000000, 0.000000000000000000, -0.000000000000000000 ) ) ;
#4460=VECTOR ( 'NONE', #5563, 1000.000000000000000 ) ;
#4461=EDGE_LOOP ( 'NONE', ( #5273, #809 ) ) ;
#4462=EDGE_CURVE ( 'NONE', #6373, #1903, #6497, .T. ) ;
#4465=ORIENTED_EDGE ( 'NONE', *, *, #8865, .F. ) ;
#4470=CARTESIAN_POINT ( 'NONE',  ( -2.293506896408097795, 80.56966535057935630, -20.00000000000000711 ) ) ;
#4472=CARTESIAN_POINT ( 'NONE',  ( 23.15769640663940265, -135.1457019118818721, -48.00000000000002132 ) ) ;
#4473=EDGE_LOOP ( 'NONE', ( #7603, #4700 ) ) ;
#4474=CARTESIAN_POINT ( 'NONE',  ( -2.293506896408097795, 120.5696653505793705, 20.00000000000000711 ) ) ;
#4475=AXIS2_PLACEMENT_3D ( 'NONE', #9689, #3213, #9906 ) ;
#4476=DIRECTION ( 'NONE',  ( -1.000000000000000000, 0.000000000000000000, -8.379529552680125332E-16 ) ) ;
#4477=CARTESIAN_POINT ( 'NONE',  ( 23.15769640663940265, -133.1457019118818721, -48.00000000000002132 ) ) ;
#4479=CARTESIAN_POINT ( 'NONE',  ( 0.000000000000000000, -135.1457019118818721, 49.99999999999997868 ) ) ;
#4480=CYLINDRICAL_SURFACE ( 'NONE', #3284, 2.000000000000001776 ) ;
#4481=CARTESIAN_POINT ( 'NONE',  ( -40.00000000000001421, -135.1457019118818721, -40.00000000000002132 ) ) ;
#4483=ORIENTED_EDGE ( 'NONE', *, *, #7033, .F. ) ;
#4485=ORIENTED_EDGE ( 'NONE', *, *, #3788, .F. ) ;
#4486=EDGE_LOOP ( 'NONE', ( #1155, #6410, #7621, #8203 ) ) ;
#4493=ORIENTED_EDGE ( 'NONE', *, *, #1904, .F. ) ;
#4494=CARTESIAN_POINT ( 'NONE',  ( 39.99999999999997158, -135.1457019118818721, 35.97499999999998010 ) ) ;
#4497=CARTESIAN_POINT ( 'NONE',  ( 25.15769640663940265, -115.1457019118818863, -48.00000000000002132 ) ) ;
#4499=EDGE_LOOP ( 'NONE', ( #9434, #6351, #1186 ) ) ;
#4503=AXIS2_PLACEMENT_3D ( 'NONE', #10274, #5491, #1474 ) ;
#4504=EDGE_CURVE ( 'NONE', #2069, #8, #437, .T. ) ;
#4506=DIRECTION ( 'NONE',  ( 1.000000000000000000, 0.000000000000000000, 0.000000000000000000 ) ) ;
#4527=VECTOR ( 'NONE', #3246, 1000.000000000000000 ) ;
#4529=CIRCLE ( 'NONE', #10458, 4.000000000000000000 ) ;
#4530=ORIENTED_EDGE ( 'NONE', *, *, #8937, .F. ) ;
#4533=CYLINDRICAL_SURFACE ( 'NONE', #4303, 7.525240063345735919 ) ;
#4536=VERTEX_POINT ( 'NONE', #10066 ) ;
#4537=CYLINDRICAL_SURFACE ( 'NONE', #9696, 10.00000000000000178 ) ;
#4539=ORIENTED_EDGE ( 'NONE', *, *, #7165, .F. ) ;
#4549=CIRCLE ( 'NONE', #8270, 26.75575292317714116 ) ;
#4551=EDGE_CURVE ( 'NONE', #1811, #8738, #2631, .T. ) ;
#4556=CARTESIAN_POINT ( 'NONE',  ( -50.00000000000002842, -135.1457019118818721, 26.62179802177713484 ) ) ;
#4562=ADVANCED_FACE ( 'NONE', ( #7149 ), #4597, .F. ) ;
#4563=ADVANCED_FACE ( 'NONE', ( #6395 ), #3965, .F. ) ;
#4565=VERTEX_POINT ( 'NONE', #8034 ) ;
#4567=VERTEX_POINT ( 'NONE', #2324 ) ;
#4568=ORIENTED_EDGE ( 'NONE', *, *, #8109, .T. ) ;
#4570=DIRECTION ( 'NONE',  ( -1.396588258780021135E-16, -0.000000000000000000, 1.000000000000000000 ) ) ;
#4571=CARTESIAN_POINT ( 'NONE',  ( 14.70649310359190309, 120.5696653505793705, 24.00000000000000711 ) ) ;
#4572=FACE_OUTER_BOUND ( 'NONE', #8518, .T. ) ;
#4573=DIRECTION ( 'NONE',  ( 1.000000000000000000, 0.000000000000000000, 0.000000000000000000 ) ) ;
#4574=ADVANCED_FACE ( 'NONE', ( #681 ), #1107, .F. ) ;
#4575=ORIENTED_EDGE ( 'NONE', *, *, #10218, .F. ) ;
#4580=DIRECTION ( 'NONE',  ( -0.6585271261848805180, 0.7525569905852198538, 0.000000000000000000 ) ) ;
#4581=PLANE ( 'NONE',  #4828 ) ;
#4582=ORIENTED_EDGE ( 'NONE', *, *, #7423, .T. ) ;
#4584=FACE_OUTER_BOUND ( 'NONE', #4280, .T. ) ;
#4585=VERTEX_POINT ( 'NONE', #7045 ) ;
#4588=CARTESIAN_POINT ( 'NONE',  ( 42.22511195853866184, 52.77167129626698028, -30.00000000000000355 ) ) ;
#4592=ORIENTED_EDGE ( 'NONE', *, *, #6735, .F. ) ;
#4593=CYLINDRICAL_SURFACE ( 'NONE', #4503, 2.000000000000001776 ) ;
#4597=CYLINDRICAL_SURFACE ( 'NONE', #8726, 2.000000000000001776 ) ;
#4598=DIRECTION ( 'NONE',  ( 0.000000000000000000, -1.000000000000000000, 0.000000000000000000 ) ) ;
#4600=CIRCLE ( 'NONE', #2566, 4.999999999999997335 ) ;
#4601=AXIS2_PLACEMENT_3D ( 'NONE', #8586, #5983, #5928 ) ;
#4607=PLANE ( 'NONE',  #4927 ) ;
#4609=VECTOR ( 'NONE', #9583, 1000.000000000000000 ) ;
#4610=CARTESIAN_POINT ( 'NONE',  ( 27.15769640663936713, -133.1457019118818721, 27.15769640663938489 ) ) ;
#4615=VECTOR ( 'NONE', #5524, 1000.000000000000000 ) ;
#4619=CARTESIAN_POINT ( 'NONE',  ( 37.59878849545336976, 32.08684478514406635, 30.00000000000000355 ) ) ;
#4622=DIRECTION ( 'NONE',  ( 0.000000000000000000, 1.000000000000000000, -0.000000000000000000 ) ) ;
#4626=EDGE_LOOP ( 'NONE', ( #4949, #9246, #4230, #8173 ) ) ;
#4627=DIRECTION ( 'NONE',  ( -1.000000000000000000, -0.000000000000000000, -0.000000000000000000 ) ) ;
#4629=AXIS2_PLACEMENT_3D ( 'NONE', #1848, #6614, #5817 ) ;
#4630=ORIENTED_EDGE ( 'NONE', *, *, #3540, .F. ) ;
#4631=EDGE_CURVE ( 'NONE', #5630, #9939, #5501, .T. ) ;
#4638=VECTOR ( 'NONE', #8677, 1000.000000000000000 ) ;
#4640=DIRECTION ( 'NONE',  ( 1.000000000000000000, 1.277197683604454965E-16, -0.000000000000000000 ) ) ;
#4646=EDGE_CURVE ( 'NONE', #8095, #5671, #5834, .T. ) ;
#4647=ORIENTED_EDGE ( 'NONE', *, *, #4331, .F. ) ;
#4649=DIRECTION ( 'NONE',  ( -0.000000000000000000, -0.000000000000000000, -1.000000000000000000 ) ) ;
#4653=CARTESIAN_POINT ( 'NONE',  ( 53.40242741783141156, 52.77167129626698028, 25.00000000000000000 ) ) ;
#4654=CARTESIAN_POINT ( 'NONE',  ( 39.99999999999997158, -145.1457019118819005, 39.99999999999997868 ) ) ;
#4655=EDGE_CURVE ( 'NONE', #640, #5617, #7536, .T. ) ;
#4658=DIRECTION ( 'NONE',  ( 0.000000000000000000, 0.000000000000000000, 1.000000000000000000 ) ) ;
#4659=VECTOR ( 'NONE', #2335, 1000.000000000000000 ) ;
#4660=EDGE_LOOP ( 'NONE', ( #1829, #9369, #7787, #2122 ) ) ;
#4663=DIRECTION ( 'NONE',  ( 0.000000000000000000, 0.000000000000000000, -1.000000000000000000 ) ) ;
#4669=ORIENTED_EDGE ( 'NONE', *, *, #8123, .T. ) ;
#4672=ORIENTED_EDGE ( 'NONE', *, *, #1932, .T. ) ;
#4673=ORIENTED_EDGE ( 'NONE', *, *, #2170, .F. ) ;
#4674=( BOUNDED_CURVE ( )  B_SPLINE_CURVE ( 3, ( #4170, #4853, #8090, #3427 ),
 .UNSPECIFIED., .F., .T. ) 
 B_SPLINE_CURVE_WITH_KNOTS ( ( 4, 4 ),
 ( 1.570796326794896558, 3.141592653589795781 ),
 .UNSPECIFIED. ) 
 CURVE ( )  GEOMETRIC_REPRESENTATION_ITEM ( )  RATIONAL_B_SPLINE_CURVE ( ( 1.000000000000000000, 0.8047378541243643824, 0.8047378541243643824, 1.000000000000000000 ) ) 
 REPRESENTATION_ITEM ( '' )  );
#4675=DIRECTION ( 'NONE',  ( -1.277197683604454965E-16, 1.000000000000000000, 0.000000000000000000 ) ) ;
#4680=FACE_OUTER_BOUND ( 'NONE', #10394, .T. ) ;
#4684=ADVANCED_FACE ( 'NONE', ( #7986 ), #8297, .F. ) ;
#4685=VECTOR ( 'NONE', #2640, 1000.000000000000000 ) ;
#4689=CARTESIAN_POINT ( 'NONE',  ( 49.99999999999998579, -145.1457019118819005, -40.00000000000002132 ) ) ;
#4691=CARTESIAN_POINT ( 'NONE',  ( 37.22511195853868315, -116.6161171811496331, 25.10513196898123311 ) ) ;
#4692=AXIS2_PLACEMENT_3D ( 'NONE', #9940, #9886, #1763 ) ;
#4695=ADVANCED_FACE ( 'NONE', ( #151 ), #4223, .F. ) ;
#4699=DIRECTION ( 'NONE',  ( 0.000000000000000000, 0.000000000000000000, 1.000000000000000000 ) ) ;
#4700=ORIENTED_EDGE ( 'NONE', *, *, #4050, .T. ) ;
#4703=CARTESIAN_POINT ( 'NONE',  ( 2.275687196221498316E-14, -133.1457019118818721, -27.15769640663941686 ) ) ;
#4705=DIRECTION ( 'NONE',  ( 0.000000000000000000, -1.000000000000000000, 0.000000000000000000 ) ) ;
#4706=DIRECTION ( 'NONE',  ( -0.000000000000000000, -0.000000000000000000, -1.000000000000000000 ) ) ;
#4709=EDGE_CURVE ( 'NONE', #8369, #5250, #271, .T. ) ;
#4710=EDGE_CURVE ( 'NONE', #847, #4386, #1113, .T. ) ;
#4711=ORIENTED_EDGE ( 'NONE', *, *, #4215, .F. ) ;
#4714=ORIENTED_EDGE ( 'NONE', *, *, #4154, .T. ) ;
#4715=CARTESIAN_POINT ( 'NONE',  ( 23.15769640663936713, -133.1457019118818721, 47.99999999999997868 ) ) ;
#4719=DIRECTION ( 'NONE',  ( -1.000000000000000000, -0.000000000000000000, -0.000000000000000000 ) ) ;
#4720=ORIENTED_EDGE ( 'NONE', *, *, #6789, .F. ) ;
#4722=VERTEX_POINT ( 'NONE', #6442 ) ;
#4723=DIRECTION ( 'NONE',  ( 0.000000000000000000, 0.000000000000000000, 1.000000000000000000 ) ) ;
#4724=EDGE_CURVE ( 'NONE', #581, #3561, #3483, .T. ) ;
#4728=CARTESIAN_POINT ( 'NONE',  ( -27.15769640663939555, -133.1457019118818721, -27.15769640663944173 ) ) ;
#4730=DIRECTION ( 'NONE',  ( -0.000000000000000000, -0.000000000000000000, -1.000000000000000000 ) ) ;
#4732=CARTESIAN_POINT ( 'NONE',  ( -48.00000000000002132, -135.1457019118818721, 27.15769640663938489 ) ) ;
#4734=CARTESIAN_POINT ( 'NONE',  ( 23.15769640663940265, -133.1457019118818721, -50.00000000000002132 ) ) ;
#4735=CYLINDRICAL_SURFACE ( 'NONE', #7210, 4.999999999999997335 ) ;
#4737=CARTESIAN_POINT ( 'NONE',  ( -48.00000000000002132, -133.1457019118818721, -23.15769640663945594 ) ) ;
#4741=DIRECTION ( 'NONE',  ( 1.000000000000000000, 0.000000000000000000, 0.000000000000000000 ) ) ;
#4742=EDGE_CURVE ( 'NONE', #2698, #9534, #5007, .T. ) ;
#4743=ADVANCED_FACE ( 'NONE', ( #6658 ), #3315, .F. ) ;
#4744=EDGE_CURVE ( 'NONE', #1800, #7344, #5855, .T. ) ;
#4745=CARTESIAN_POINT ( 'NONE',  ( 14.70649310359190309, 80.56966535057935630, 20.00000000000000711 ) ) ;
#4746=VECTOR ( 'NONE', #9378, 1000.000000000000000 ) ;
#4747=DIRECTION ( 'NONE',  ( 0.6585271261848814062, -0.7525569905852189656, -6.854174792162727679E-16 ) ) ;
#4749=SPHERICAL_SURFACE ( 'NONE', #3067, 2.000000000000000000 ) ;
#4750=FACE_OUTER_BOUND ( 'NONE', #10193, .T. ) ;
#4751=ORIENTED_EDGE ( 'NONE', *, *, #10279, .T. ) ;
#4752=CARTESIAN_POINT ( 'NONE',  ( 59.99999999999999289, -145.1457019118819005, -30.00000000000000355 ) ) ;
#4754=DIRECTION ( 'NONE',  ( -0.000000000000000000, 1.000000000000000000, 0.000000000000000000 ) ) ;
#4755=DIRECTION ( 'NONE',  ( -0.000000000000000000, 1.000000000000000000, -0.000000000000000000 ) ) ;
#4758=VERTEX_POINT ( 'NONE', #9692 ) ;
#4759=PLANE ( 'NONE',  #564 ) ;
#4764=ORIENTED_EDGE ( 'NONE', *, *, #8508, .F. ) ;
#4766=CIRCLE ( 'NONE', #8330, 5.000000000000001776 ) ;
#4767=ORIENTED_EDGE ( 'NONE', *, *, #2654, .F. ) ;
#4768=AXIS2_PLACEMENT_3D ( 'NONE', #7615, #10161, #3639 ) ;
#4772=CARTESIAN_POINT ( 'NONE',  ( -24.41866285951199345, -134.3099192498708874, -50.00000000000002132 ) ) ;
#4776=VERTEX_POINT ( 'NONE', #42 ) ;
#4777=AXIS2_PLACEMENT_3D ( 'NONE', #6870, #5225, #7771 ) ;
#4778=DIRECTION ( 'NONE',  ( 0.000000000000000000, 1.000000000000000000, 0.000000000000000000 ) ) ;
#4779=EDGE_CURVE ( 'NONE', #7038, #415, #4900, .T. ) ;
#4780=ORIENTED_EDGE ( 'NONE', *, *, #5334, .F. ) ;
#4782=DIRECTION ( 'NONE',  ( -0.000000000000000000, 1.000000000000000000, -0.000000000000000000 ) ) ;
#4784=DIRECTION ( 'NONE',  ( 6.982941293900105430E-16, 0.000000000000000000, -1.000000000000000000 ) ) ;
#4785=CARTESIAN_POINT ( 'NONE',  ( 4.856471286862176662, 145.0444252872335937, 12.50000000000000355 ) ) ;
#4787=DIRECTION ( 'NONE',  ( 0.000000000000000000, 0.000000000000000000, 1.000000000000000000 ) ) ;
#4794=AXIS2_PLACEMENT_3D ( 'NONE', #6657, #5694, #93 ) ;
#4795=DIRECTION ( 'NONE',  ( 1.000000000000000000, -0.000000000000000000, 8.379529552680125332E-16 ) ) ;
#4796=LINE ( 'NONE', #3754, #4638 ) ;
#4800=DIRECTION ( 'NONE',  ( 0.9973063064792990762, 0.07334937666141773394, 0.000000000000000000 ) ) ;
#4804=CARTESIAN_POINT ( 'NONE',  ( -18.34874108452141783, -140.1746510883711778, -24.43989726270230634 ) ) ;
#4805=ORIENTED_EDGE ( 'NONE', *, *, #9679, .F. ) ;
#4807=CARTESIAN_POINT ( 'NONE',  ( 17.97972049165455388, 37.08684478514405214, 12.50000000000000000 ) ) ;
#4809=DIRECTION ( 'NONE',  ( 0.000000000000000000, 0.000000000000000000, -1.000000000000000000 ) ) ;
#4810=AXIS2_PLACEMENT_3D ( 'NONE', #6617, #165, #8954 ) ;
#4811=DIRECTION ( 'NONE',  ( -0.000000000000000000, 1.000000000000000000, 0.000000000000000000 ) ) ;
#4812=ORIENTED_EDGE ( 'NONE', *, *, #1709, .F. ) ;
#4814=CIRCLE ( 'NONE', #1271, 10.00000000000000178 ) ;
#4817=EDGE_CURVE ( 'NONE', #3545, #9491, #5321, .T. ) ;
#4818=EDGE_LOOP ( 'NONE', ( #4925, #3116, #1992, #10022, #4384, #7366, #8181, #5976, #9709, #7827, #4879, #5831, #3158, #4972, #7380, #6621 ) ) ;
#4821=AXIS2_PLACEMENT_3D ( 'NONE', #7730, #473, #8787 ) ;
#4822=CARTESIAN_POINT ( 'NONE',  ( -27.15769640663940976, -133.1457019118818721, 25.15769640663938134 ) ) ;
#4825=FACE_OUTER_BOUND ( 'NONE', #5079, .T. ) ;
#4826=VERTEX_POINT ( 'NONE', #8405 ) ;
#4828=AXIS2_PLACEMENT_3D ( 'NONE', #2144, #612, #10320 ) ;
#4829=EDGE_CURVE ( 'NONE', #7484, #5250, #9959, .T. ) ;
#4833=AXIS2_PLACEMENT_3D ( 'NONE', #2050, #5915, #9155 ) ;
#4834=CARTESIAN_POINT ( 'NONE',  ( -38.19229777560033057, -43.28483205141633761, -12.50000000000000000 ) ) ;
#4838=CARTESIAN_POINT ( 'NONE',  ( -27.15769640663939199, -135.1457019118818721, -27.15769640663944173 ) ) ;
#4839=ORIENTED_EDGE ( 'NONE', *, *, #10056, .F. ) ;
#4841=AXIS2_PLACEMENT_3D ( 'NONE', #8440, #6157, #6853 ) ;
#4842=ORIENTED_EDGE ( 'NONE', *, *, #1643, .F. ) ;
#4846=ADVANCED_FACE ( 'NONE', ( #1990 ), #2089, .T. ) ;
#4847=AXIS2_PLACEMENT_3D ( 'NONE', #8413, #10219, #6019 ) ;
#4848=DIRECTION ( 'NONE',  ( 0.000000000000000000, 0.000000000000000000, -1.000000000000000000 ) ) ;
#4851=CARTESIAN_POINT ( 'NONE',  ( 27.15769640663938489, -133.1457019118818721, -25.15769640663940621 ) ) ;
#4853=CARTESIAN_POINT ( 'NONE',  ( 97.72361618343359169, -145.1457019118819005, -30.00000000000000711 ) ) ;
#4860=DIRECTION ( 'NONE',  ( -0.7367503238654704578, 0.6761648913424330720, -0.000000000000000000 ) ) ;
#4861=CARTESIAN_POINT ( 'NONE',  ( 27.15769640663936713, -117.1457019118819005, 27.15769640663938489 ) ) ;
#4866=LINE ( 'NONE', #8101, #7363 ) ;
#4868=ORIENTED_EDGE ( 'NONE', *, *, #7098, .T. ) ;
#4870=AXIS2_PLACEMENT_3D ( 'NONE', #641, #4754, #10441 ) ;
#4871=VERTEX_POINT ( 'NONE', #2780 ) ;
#4878=EDGE_CURVE ( 'NONE', #6462, #2154, #4382, .T. ) ;
#4879=ORIENTED_EDGE ( 'NONE', *, *, #5146, .T. ) ;
#4884=EDGE_LOOP ( 'NONE', ( #1547, #336, #18, #2877 ) ) ;
#4885=DIRECTION ( 'NONE',  ( 0.000000000000000000, 0.000000000000000000, 1.000000000000000000 ) ) ;
#4886=DIRECTION ( 'NONE',  ( 1.396588258780021135E-16, -0.000000000000000000, 1.000000000000000000 ) ) ;
#4887=DIRECTION ( 'NONE',  ( 0.000000000000000000, -1.000000000000000000, 0.000000000000000000 ) ) ;
#4888=ADVANCED_FACE ( 'NONE', ( #3636 ), #6011, .F. ) ;
#4889=AXIS2_PLACEMENT_3D ( 'NONE', #337, #8434, #7535 ) ;
#4895=ORIENTED_EDGE ( 'NONE', *, *, #1456, .F. ) ;
#4896=CARTESIAN_POINT ( 'NONE',  ( -24.41868145091758535, -134.3099331815685105, 49.99999999999998579 ) ) ;
#4897=ORIENTED_EDGE ( 'NONE', *, *, #1799, .F. ) ;
#4900=LINE ( 'NONE', #2418, #7893 ) ;
#4901=CARTESIAN_POINT ( 'NONE',  ( 4.856471286862175774, 147.5696653505793279, -25.00000000000000355 ) ) ;
#4904=ORIENTED_EDGE ( 'NONE', *, *, #4779, .F. ) ;
#4905=CARTESIAN_POINT ( 'NONE',  ( -40.00000000000001421, -135.1707019118818778, -40.00000000000002132 ) ) ;
#4906=CARTESIAN_POINT ( 'NONE',  ( 85.07264007511442117, 55.10093597859600578, 25.00000000000000000 ) ) ;
#4907=DIRECTION ( 'NONE',  ( -1.396588258780021135E-16, 0.000000000000000000, 1.000000000000000000 ) ) ;
#4908=CARTESIAN_POINT ( 'NONE',  ( 0.000000000000000000, -117.1457019118819005, 47.99999999999997868 ) ) ;
#4912=VERTEX_POINT ( 'NONE', #9359 ) ;
#4913=ORIENTED_EDGE ( 'NONE', *, *, #2682, .F. ) ;
#4914=TOROIDAL_SURFACE ( 'NONE', #3923, 4.000000000000000000, 2.000000000000000000 ) ;
#4915=ORIENTED_EDGE ( 'NONE', *, *, #5104, .F. ) ;
#4917=EDGE_LOOP ( 'NONE', ( #6767, #1018 ) ) ;
#4920=AXIS2_PLACEMENT_3D ( 'NONE', #7339, #4159, #5636 ) ;
#4925=ORIENTED_EDGE ( 'NONE', *, *, #2549, .F. ) ;
#4927=AXIS2_PLACEMENT_3D ( 'NONE', #531, #5453, #587 ) ;
#4936=DIRECTION ( 'NONE',  ( -0.6585271261848796298, 0.7525569905852207420, 0.000000000000000000 ) ) ;
#4941=DIRECTION ( 'NONE',  ( 0.000000000000000000, 0.000000000000000000, 1.000000000000000000 ) ) ;
#4948=VECTOR ( 'NONE', #1825, 1000.000000000000000 ) ;
#4949=ORIENTED_EDGE ( 'NONE', *, *, #9190, .F. ) ;
#4952=DIRECTION ( 'NONE',  ( 0.000000000000000000, 0.000000000000000000, 1.000000000000000000 ) ) ;
#4955=DIRECTION ( 'NONE',  ( 0.000000000000000000, 1.000000000000000000, 0.000000000000000000 ) ) ;
#4958=DIRECTION ( 'NONE',  ( 1.277197683604454965E-16, -1.000000000000000000, 0.000000000000000000 ) ) ;
#4961=DIRECTION ( 'NONE',  ( -0.000000000000000000, -1.000000000000000000, -0.000000000000000000 ) ) ;
#4963=ORIENTED_EDGE ( 'NONE', *, *, #7689, .F. ) ;
#4965=DIRECTION ( 'NONE',  ( 0.000000000000000000, -1.000000000000000000, 0.000000000000000000 ) ) ;
#4966=ADVANCED_FACE ( 'NONE', ( #9581 ), #3099, .T. ) ;
#4968=LINE ( 'NONE', #5077, #1779 ) ;
#4969=AXIS2_PLACEMENT_3D ( 'NONE', #9383, #2523, #2417 ) ;
#4971=ORIENTED_EDGE ( 'NONE', *, *, #1959, .F. ) ;
#4972=ORIENTED_EDGE ( 'NONE', *, *, #3776, .F. ) ;
#4973=CARTESIAN_POINT ( 'NONE',  ( -38.19229777560033057, 37.08684478514405214, -12.50000000000000000 ) ) ;
#4976=CARTESIAN_POINT ( 'NONE',  ( 23.76520584195949226, -145.1457019118819005, -50.00000000000002132 ) ) ;
#4978=DIRECTION ( 'NONE',  ( 0.000000000000000000, 0.000000000000000000, -1.000000000000000000 ) ) ;
#4984=AXIS2_PLACEMENT_3D ( 'NONE', #5025, #9976, #4235 ) ;
#4992=ADVANCED_FACE ( 'NONE', ( #5376 ), #4735, .T. ) ;
#4993=FACE_OUTER_BOUND ( 'NONE', #3314, .T. ) ;
#4995=ORIENTED_EDGE ( 'NONE', *, *, #2722, .F. ) ;
#5000=CARTESIAN_POINT ( 'NONE',  ( -23.64292728780887032, -133.6309146189979060, 49.99999999999997868 ) ) ;
#5007=LINE ( 'NONE', #1622, #948 ) ;
#5008=EDGE_CURVE ( 'NONE', #8658, #6094, #5536, .T. ) ;
#5011=VECTOR ( 'NONE', #5196, 1000.000000000000000 ) ;
#5012=EDGE_CURVE ( 'NONE', #8070, #6030, #8303, .T. ) ;
#5014=ORIENTED_EDGE ( 'NONE', *, *, #10042, .F. ) ;
#5017=VERTEX_POINT ( 'NONE', #561 ) ;
#5019=CARTESIAN_POINT ( 'NONE',  ( 4.856471286862175774, 152.5696653505793279, 30.00000000000000355 ) ) ;
#5021=AXIS2_PLACEMENT_3D ( 'NONE', #4015, #6549, #9798 ) ;
#5023=DIRECTION ( 'NONE',  ( -0.000000000000000000, 1.000000000000000000, -0.000000000000000000 ) ) ;
#5024=ADVANCED_FACE ( 'NONE', ( #1356 ), #4581, .F. ) ;
#5025=CARTESIAN_POINT ( 'NONE',  ( -27.15769640663941331, -133.1457019118818721, 27.15769640663938489 ) ) ;
#5026=VECTOR ( 'NONE', #10206, 1000.000000000000000 ) ;
#5028=B_SPLINE_CURVE_WITH_KNOTS ( 'NONE', 3,
 ( #4734, #6381, #9466, #8772, #1298, #1515, #611, #560, #7973, #714 ),
 .UNSPECIFIED., .F., .F.,
 ( 4, 2, 2, 2, 4 ),
 ( -8.944271910636758738E-06, 0.001019331502940711920, 0.002047607277792060521, 0.003075883052643409339, 0.004104158827494757723 ),
 .UNSPECIFIED. ) ;
#5029=EDGE_LOOP ( 'NONE', ( #8827, #6816 ) ) ;
#5030=VERTEX_POINT ( 'NONE', #3795 ) ;
#5033=AXIS2_PLACEMENT_3D ( 'NONE', #4619, #7855, #6519 ) ;
#5035=DIRECTION ( 'NONE',  ( 1.000000000000000000, 0.000000000000000000, -0.000000000000000000 ) ) ;
#5036=EDGE_LOOP ( 'NONE', ( #6393, #7969, #5560, #10029 ) ) ;
#5037=DIRECTION ( 'NONE',  ( 0.000000000000000000, -1.000000000000000000, 0.000000000000000000 ) ) ;
#5040=AXIS2_PLACEMENT_3D ( 'NONE', #329, #9168, #6729 ) ;
#5043=CIRCLE ( 'NONE', #485, 2.000000000000001776 ) ;
#5050=DIRECTION ( 'NONE',  ( 0.000000000000000000, 0.000000000000000000, -1.000000000000000000 ) ) ;
#5053=CYLINDRICAL_SURFACE ( 'NONE', #6138, 3.297986701801175258 ) ;
#5056=LINE ( 'NONE', #87, #3711 ) ;
#5060=CARTESIAN_POINT ( 'NONE',  ( 99.80027788547049283, -145.1457019118819005, 25.00000000000000000 ) ) ;
#5061=CARTESIAN_POINT ( 'NONE',  ( -21.44003972449636208, -143.0117419471019673, -6.332076144530982553 ) ) ;
#5066=VERTEX_POINT ( 'NONE', #8664 ) ;
#5069=EDGE_CURVE ( 'NONE', #1149, #6373, #3905, .T. ) ;
#5072=CARTESIAN_POINT ( 'NONE',  ( 1.940506014114293224E-14, -117.1457019118819005, -23.15769640663941331 ) ) ;
#5073=DIRECTION ( 'NONE',  ( 0.000000000000000000, 1.000000000000000000, 0.000000000000000000 ) ) ;
#5074=DIRECTION ( 'NONE',  ( 0.000000000000000000, 0.000000000000000000, -1.000000000000000000 ) ) ;
#5077=CARTESIAN_POINT ( 'NONE',  ( 25.15769640663937778, -115.1457019118818863, -23.15769640663940976 ) ) ;
#5079=EDGE_LOOP ( 'NONE', ( #6218, #2387, #8316, #8023 ) ) ;
#5081=ADVANCED_FACE ( 'NONE', ( #4993 ), #6198, .F. ) ;
#5082=EDGE_CURVE ( 'NONE', #1253, #5224, #82, .T. ) ;
#5085=ORIENTED_EDGE ( 'NONE', *, *, #8829, .T. ) ;
#5090=AXIS2_PLACEMENT_3D ( 'NONE', #3871, #5600, #1577 ) ;
#5091=ORIENTED_EDGE ( 'NONE', *, *, #3218, .T. ) ;
#5096=EDGE_CURVE ( 'NONE', #7140, #2630, #7215, .T. ) ;
#5098=ORIENTED_EDGE ( 'NONE', *, *, #5667, .F. ) ;
#5099=LINE ( 'NONE', #4305, #7399 ) ;
#5104=EDGE_CURVE ( 'NONE', #5655, #898, #3200, .T. ) ;
#5106=AXIS2_PLACEMENT_3D ( 'NONE', #3736, #4778, #6965 ) ;
#5110=DIRECTION ( 'NONE',  ( -0.000000000000000000, 1.000000000000000000, -0.000000000000000000 ) ) ;
#5111=VERTEX_POINT ( 'NONE', #4838 ) ;
#5114=CIRCLE ( 'NONE', #549, 7.500000000000000000 ) ;
#5115=AXIS2_PLACEMENT_3D ( 'NONE', #10420, #7820, #4787 ) ;
#5116=DIRECTION ( 'NONE',  ( -0.000000000000000000, -1.000000000000000000, -0.000000000000000000 ) ) ;
#5123=EDGE_LOOP ( 'NONE', ( #9060, #1585, #159, #8172 ) ) ;
#5125=ORIENTED_EDGE ( 'NONE', *, *, #414, .F. ) ;
#5130=FACE_OUTER_BOUND ( 'NONE', #5580, .T. ) ;
#5134=ORIENTED_EDGE ( 'NONE', *, *, #2161, .T. ) ;
#5135=ORIENTED_EDGE ( 'NONE', *, *, #6294, .T. ) ;
#5136=CIRCLE ( 'NONE', #6150, 2.000000000000001776 ) ;
#5138=CARTESIAN_POINT ( 'NONE',  ( -50.00000000000002132, -134.3099192498709158, 24.41866285951200766 ) ) ;
#5140=VECTOR ( 'NONE', #8990, 1000.000000000000000 ) ;
#5141=ORIENTED_EDGE ( 'NONE', *, *, #3206, .F. ) ;
#5144=EDGE_CURVE ( 'NONE', #5066, #5352, #974, .T. ) ;
#5146=EDGE_CURVE ( 'NONE', #9448, #9884, #6364, .T. ) ;
#5147=ORIENTED_EDGE ( 'NONE', *, *, #3218, .F. ) ;
#5148=AXIS2_PLACEMENT_3D ( 'NONE', #8558, #6974, #6168 ) ;
#5149=ORIENTED_EDGE ( 'NONE', *, *, #5381, .F. ) ;
#5152=CARTESIAN_POINT ( 'NONE',  ( 23.15769640663938134, -115.1457019118818863, -27.15769640663941686 ) ) ;
#5153=LINE ( 'NONE', #4367, #1222 ) ;
#5156=AXIS2_PLACEMENT_3D ( 'NONE', #2434, #9498, #8899 ) ;
#5157=ADVANCED_FACE ( 'NONE', ( #3252 ), #10270, .T. ) ;
#5160=ORIENTED_EDGE ( 'NONE', *, *, #10204, .F. ) ;
#5161=CARTESIAN_POINT ( 'NONE',  ( 10.51964330236497602, 150.0000000000000000, 25.00000000000000000 ) ) ;
#5163=APPLICATION_CONTEXT ( 'automotive_design' ) ;
#5165=FACE_OUTER_BOUND ( 'NONE', #2528, .T. ) ;
#5172=LINE ( 'NONE', #9208, #3505 ) ;
#5175=DIRECTION ( 'NONE',  ( -0.000000000000000000, -0.000000000000000000, -1.000000000000000000 ) ) ;
#5176=DIRECTION ( 'NONE',  ( 1.000000000000000000, 0.000000000000000000, -0.000000000000000000 ) ) ;
#5177=EDGE_LOOP ( 'NONE', ( #3106, #6299, #6172, #3913 ) ) ;
#5178=VECTOR ( 'NONE', #320, 1000.000000000000000 ) ;
#5179=LINE ( 'NONE', #2901, #3198 ) ;
#5182=AXIS2_PLACEMENT_3D ( 'NONE', #3838, #2081, #659 ) ;
#5183=CARTESIAN_POINT ( 'NONE',  ( -16.29350689640809691, -115.1457019118818863, 27.01918567566963247 ) ) ;
#5185=ORIENTED_EDGE ( 'NONE', *, *, #239, .T. ) ;
#5187=VECTOR ( 'NONE', #5037, 1000.000000000000000 ) ;
#5191=LINE ( 'NONE', #8426, #2841 ) ;
#5192=DIRECTION ( 'NONE',  ( -1.387778780781445676E-16, 0.000000000000000000, 1.000000000000000000 ) ) ;
#5193=DIRECTION ( 'NONE',  ( 0.000000000000000000, -1.000000000000000000, 0.000000000000000000 ) ) ;
#5194=VECTOR ( 'NONE', #8565, 1000.000000000000000 ) ;
#5196=DIRECTION ( 'NONE',  ( 1.000000000000000000, 0.000000000000000000, 0.000000000000000000 ) ) ;
#5201=ORIENTED_EDGE ( 'NONE', *, *, #6481, .T. ) ;
#5202=EDGE_CURVE ( 'NONE', #36, #7357, #2623, .T. ) ;
#5204=DIRECTION ( 'NONE',  ( -0.07334937666141724821, 0.9973063064792989652, 0.000000000000000000 ) ) ;
#5208=CARTESIAN_POINT ( 'NONE',  ( 6.756858349438876310, 146.7073643690755773, -25.00000000000000355 ) ) ;
#5212=ORIENTED_EDGE ( 'NONE', *, *, #7195, .T. ) ;
#5213=CARTESIAN_POINT ( 'NONE',  ( -48.00000000000002132, -117.1457019118819005, 23.15769640663938134 ) ) ;
#5214=ORIENTED_EDGE ( 'NONE', *, *, #6119, .T. ) ;
#5219=CIRCLE ( 'NONE', #7090, 2.000000000000001776 ) ;
#5221=CARTESIAN_POINT ( 'NONE',  ( 17.97972049165455388, 17.84145331825995484, -30.00000000000000355 ) ) ;
#5222=CARTESIAN_POINT ( 'NONE',  ( 37.25871876463539678, -134.3867942047928921, 25.58368939469043468 ) ) ;
#5224=VERTEX_POINT ( 'NONE', #9297 ) ;
#5225=DIRECTION ( 'NONE',  ( -1.000000000000000000, 0.000000000000000000, 0.000000000000000000 ) ) ;
#5230=VERTEX_POINT ( 'NONE', #10094 ) ;
#5231=CARTESIAN_POINT ( 'NONE',  ( 59.99999999999997868, 52.77167129626698028, 40.00000000000000000 ) ) ;
#5232=CARTESIAN_POINT ( 'NONE',  ( 23.15769640663936713, -117.1457019118819005, 49.99999999999997868 ) ) ;
#5235=DIRECTION ( 'NONE',  ( -0.000000000000000000, 0.000000000000000000, 1.000000000000000000 ) ) ;
#5237=ADVANCED_FACE ( 'NONE', ( #448 ), #7648, .T. ) ;
#5238=ADVANCED_FACE ( 'NONE', ( #5999 ), #1077, .F. ) ;
#5241=DIRECTION ( 'NONE',  ( 0.000000000000000000, 0.000000000000000000, 1.000000000000000000 ) ) ;
#5245=DIRECTION ( 'NONE',  ( 0.000000000000000000, 0.000000000000000000, 1.000000000000000000 ) ) ;
#5247=ORIENTED_EDGE ( 'NONE', *, *, #3658, .T. ) ;
#5249=CARTESIAN_POINT ( 'NONE',  ( 25.15769640663935292, -133.1457019118818721, 2.459446039362539254E-14 ) ) ;
#5250=VERTEX_POINT ( 'NONE', #10148 ) ;
#5259=AXIS2_PLACEMENT_3D ( 'NONE', #988, #9854, #1783 ) ;
#5263=FACE_OUTER_BOUND ( 'NONE', #2476, .T. ) ;
#5264=AXIS2_PLACEMENT_3D ( 'NONE', #2025, #6958, #10195 ) ;
#5265=CARTESIAN_POINT ( 'NONE',  ( 37.24329735151886211, -134.1666765793263778, 25.43275615213076790 ) ) ;
#5266=CARTESIAN_POINT ( 'NONE',  ( -23.76520584195948516, -145.1457019118819005, -97.78965767959371647 ) ) ;
#5269=DIRECTION ( 'NONE',  ( 1.000000000000000000, 0.000000000000000000, 0.000000000000000000 ) ) ;
#5270=EDGE_CURVE ( 'NONE', #7848, #6574, #2876, .T. ) ;
#5273=ORIENTED_EDGE ( 'NONE', *, *, #2171, .T. ) ;
#5275=VECTOR ( 'NONE', #4100, 1000.000000000000000 ) ;
#5277=AXIS2_PLACEMENT_3D ( 'NONE', #9927, #9876, #9119 ) ;
#5279=ORIENTED_EDGE ( 'NONE', *, *, #9553, .T. ) ;
#5280=DIRECTION ( 'NONE',  ( -1.000000000000000000, 0.000000000000000000, -8.379529552680124346E-16 ) ) ;
#5286=DIRECTION ( 'NONE',  ( -0.000000000000000000, 1.000000000000000000, -0.000000000000000000 ) ) ;
#5288=EDGE_CURVE ( 'NONE', #1218, #389, #285, .T. ) ;
#5290=ORIENTED_EDGE ( 'NONE', *, *, #2625, .T. ) ;
#5294=DIRECTION ( 'NONE',  ( 1.000000000000000000, 0.000000000000000000, 1.734723475976805517E-15 ) ) ;
#5296=CARTESIAN_POINT ( 'NONE',  ( 37.22511195853868315, -116.6161171811496189, -25.10513196898124377 ) ) ;
#5304=EDGE_CURVE ( 'NONE', #8341, #8447, #5, .T. ) ;
#5305=CARTESIAN_POINT ( 'NONE',  ( -23.15769640663940976, -117.1457019118819005, 47.99999999999997868 ) ) ;
#5312=DIRECTION ( 'NONE',  ( 0.000000000000000000, 0.000000000000000000, 1.000000000000000000 ) ) ;
#5314=AXIS2_PLACEMENT_3D ( 'NONE', #4445, #6991, #6027 ) ;
#5317=EDGE_CURVE ( 'NONE', #7162, #8567, #6705, .T. ) ;
#5319=CARTESIAN_POINT ( 'NONE',  ( 17.97972049165455388, 37.08684478514406635, 25.00000000000000000 ) ) ;
#5320=DIRECTION ( 'NONE',  ( 0.000000000000000000, 0.000000000000000000, 1.000000000000000000 ) ) ;
#5321=LINE ( 'NONE', #8559, #10426 ) ;
#5323=CIRCLE ( 'NONE', #6516, 4.000000000000000000 ) ;
#5327=DIRECTION ( 'NONE',  ( -1.396588258780021135E-16, 0.000000000000000000, -1.000000000000000000 ) ) ;
#5328=ORIENTED_EDGE ( 'NONE', *, *, #2091, .T. ) ;
#5329=AXIS2_PLACEMENT_3D ( 'NONE', #8885, #7456, #4952 ) ;
#5332=EDGE_CURVE ( 'NONE', #86, #939, #8053, .T. ) ;
#5334=EDGE_CURVE ( 'NONE', #3261, #4722, #10197, .T. ) ;
#5335=EDGE_CURVE ( 'NONE', #9948, #2404, #620, .T. ) ;
#5336=DIRECTION ( 'NONE',  ( -0.000000000000000000, 1.000000000000000000, -0.000000000000000000 ) ) ;
#5341=ORIENTED_EDGE ( 'NONE', *, *, #5727, .F. ) ;
#5345=CARTESIAN_POINT ( 'NONE',  ( -2.293506896408097795, 42.08684478514410188, 30.00000000000000355 ) ) ;
#5348=CARTESIAN_POINT ( 'NONE',  ( 14.70649310359190309, 80.56966535057935630, -20.00000000000000711 ) ) ;
#5349=( BOUNDED_CURVE ( )  B_SPLINE_CURVE ( 3, ( #5060, #8295, #1033, #4270 ),
 .UNSPECIFIED., .F., .T. ) 
 B_SPLINE_CURVE_WITH_KNOTS ( ( 4, 4 ),
 ( 0.000000000000000000, 1.570796326794896558 ),
 .UNSPECIFIED. ) 
 CURVE ( )  GEOMETRIC_REPRESENTATION_ITEM ( )  RATIONAL_B_SPLINE_CURVE ( ( 1.000000000000000000, 0.8047378541243649375, 0.8047378541243649375, 1.000000000000000000 ) ) 
 REPRESENTATION_ITEM ( '' )  );
#5352=VERTEX_POINT ( 'NONE', #9457 ) ;
#5356=ORIENTED_EDGE ( 'NONE', *, *, #10367, .T. ) ;
#5357=VERTEX_POINT ( 'NONE', #5474 ) ;
#5358=LINE ( 'NONE', #6957, #4193 ) ;
#5359=DIRECTION ( 'NONE',  ( 0.000000000000000000, 0.000000000000000000, -1.000000000000000000 ) ) ;
#5361=DIRECTION ( 'NONE',  ( 0.000000000000000000, -0.000000000000000000, 1.000000000000000000 ) ) ;
#5363=CIRCLE ( 'NONE', #795, 10.00000000000000178 ) ;
#5364=FACE_BOUND ( 'NONE', #8873, .T. ) ;
#5365=ORIENTED_EDGE ( 'NONE', *, *, #5012, .T. ) ;
#5367=EDGE_CURVE ( 'NONE', #8901, #4776, #2191, .T. ) ;
#5376=FACE_OUTER_BOUND ( 'NONE', #1705, .T. ) ;
#5381=EDGE_CURVE ( 'NONE', #5111, #6261, #2814, .T. ) ;
#5385=ORIENTED_EDGE ( 'NONE', *, *, #6575, .T. ) ;
#5386=AXIS2_PLACEMENT_3D ( 'NONE', #6389, #9642, #2318 ) ;
#5390=CARTESIAN_POINT ( 'NONE',  ( -18.34874108452141783, -140.1746510883711778, 7.212905963064383918 ) ) ;
#5393=CARTESIAN_POINT ( 'NONE',  ( 26.62179802177712062, -135.1457019118818721, 49.99999999999997868 ) ) ;
#5395=ADVANCED_FACE ( 'NONE', ( #5521 ), #1505, .T. ) ;
#5397=EDGE_CURVE ( 'NONE', #3840, #3587, #499, .T. ) ;
#5398=CYLINDRICAL_SURFACE ( 'NONE', #2138, 3.999999999999989786 ) ;
#5399=ADVANCED_FACE ( 'NONE', ( #6963 ), #6269, .F. ) ;
#5402=CARTESIAN_POINT ( 'NONE',  ( -18.34874108452141783, -140.1746510883711778, -97.78965767959371647 ) ) ;
#5405=CARTESIAN_POINT ( 'NONE',  ( -2.293506896408097795, 120.5696653505793705, 20.00000000000000711 ) ) ;
#5406=DIRECTION ( 'NONE',  ( -0.000000000000000000, 1.000000000000000000, -0.000000000000000000 ) ) ;
#5408=ORIENTED_EDGE ( 'NONE', *, *, #500, .T. ) ;
#5409=EDGE_CURVE ( 'NONE', #6945, #3453, #9250, .T. ) ;
#5413=ORIENTED_EDGE ( 'NONE', *, *, #5202, .F. ) ;
#5415=CARTESIAN_POINT ( 'NONE',  ( 23.15769640663936713, -133.1457019118818721, 49.99999999999997868 ) ) ;
#5418=DIRECTION ( 'NONE',  ( -1.000000000000000000, 0.000000000000000000, 0.000000000000000000 ) ) ;
#5425=EDGE_CURVE ( 'NONE', #8668, #7191, #6217, .T. ) ;
#5426=CARTESIAN_POINT ( 'NONE',  ( -18.34874108452141783, -140.1746510883711778, -50.00000000000002132 ) ) ;
#5430=CIRCLE ( 'NONE', #700, 31.75575292317714471 ) ;
#5431=LINE ( 'NONE', #10370, #8502 ) ;
#5437=AXIS2_PLACEMENT_3D ( 'NONE', #6431, #924, #9033 ) ;
#5438=AXIS2_PLACEMENT_3D ( 'NONE', #9311, #1145, #1248 ) ;
#5439=VERTEX_POINT ( 'NONE', #2134 ) ;
#5440=DIRECTION ( 'NONE',  ( -0.000000000000000000, 1.000000000000000000, -0.000000000000000000 ) ) ;
#5441=ADVANCED_FACE ( 'NONE', ( #4680, #5364 ), #8603, .F. ) ;
#5443=CARTESIAN_POINT ( 'NONE',  ( 6.756858349438874534, 146.7073643690755773, 25.00000000000000000 ) ) ;
#5445=CARTESIAN_POINT ( 'NONE',  ( 4.856471286862176662, 147.5696653505793279, -25.00000000000002132 ) ) ;
#5446=DIRECTION ( 'NONE',  ( -0.000000000000000000, -1.000000000000000000, -0.000000000000000000 ) ) ;
#5447=CIRCLE ( 'NONE', #5106, 10.00000000000000178 ) ;
#5450=DIRECTION ( 'NONE',  ( 1.000000000000000000, -0.000000000000000000, 8.379529552680125332E-16 ) ) ;
#5453=DIRECTION ( 'NONE',  ( 1.000000000000000000, 0.000000000000000000, -0.000000000000000000 ) ) ;
#5454=AXIS2_PLACEMENT_3D ( 'NONE', #4337, #6131, #6720 ) ;
#5455=ORIENTED_EDGE ( 'NONE', *, *, #4551, .F. ) ;
#5456=CIRCLE ( 'NONE', #6304, 2.000000000000001776 ) ;
#5457=LINE ( 'NONE', #7058, #4460 ) ;
#5462=ORIENTED_EDGE ( 'NONE', *, *, #9293, .T. ) ;
#5464=CIRCLE ( 'NONE', #9515, 4.000000000000000000 ) ;
#5467=FACE_BOUND ( 'NONE', #3191, .T. ) ;
#5472=ADVANCED_FACE ( 'NONE', ( #70 ), #8115, .F. ) ;
#5474=CARTESIAN_POINT ( 'NONE',  ( 23.15769640663939910, -115.1457019118818863, -48.00000000000002132 ) ) ;
#5476=ORIENTED_EDGE ( 'NONE', *, *, #6543, .T. ) ;
#5479=CARTESIAN_POINT ( 'NONE',  ( 14.70649310359190309, 80.56966535057935630, -16.00000000000000711 ) ) ;
#5480=CARTESIAN_POINT ( 'NONE',  ( 53.40242741783141156, 52.77167129626698028, -25.00000000000000355 ) ) ;
#5482=VECTOR ( 'NONE', #4116, 1000.000000000000000 ) ;
#5483=ORIENTED_EDGE ( 'NONE', *, *, #10298, .F. ) ;
#5484=DIRECTION ( 'NONE',  ( 0.000000000000000000, 0.000000000000000000, 1.000000000000000000 ) ) ;
#5487=DIRECTION ( 'NONE',  ( -0.000000000000000000, -0.000000000000000000, 1.000000000000000000 ) ) ;
#5488=EDGE_LOOP ( 'NONE', ( #747, #8066 ) ) ;
#5489=AXIS2_PLACEMENT_3D ( 'NONE', #2564, #4784, #5793 ) ;
#5490=VERTEX_POINT ( 'NONE', #7224 ) ;
#5491=DIRECTION ( 'NONE',  ( 0.000000000000000000, 1.000000000000000000, 0.000000000000000000 ) ) ;
#5493=DIRECTION ( 'NONE',  ( 0.000000000000000000, 0.000000000000000000, -1.000000000000000000 ) ) ;
#5494=CARTESIAN_POINT ( 'NONE',  ( 39.99999999999997158, -135.1457019118818721, 44.02499999999997726 ) ) ;
#5496=DIRECTION ( 'NONE',  ( 0.000000000000000000, 1.000000000000000000, 0.000000000000000000 ) ) ;
#5498=VECTOR ( 'NONE', #5406, 1000.000000000000000 ) ;
#5501=CIRCLE ( 'NONE', #930, 2.000000000000001776 ) ;
#5503=ORIENTED_EDGE ( 'NONE', *, *, #1846, .T. ) ;
#5504=FACE_OUTER_BOUND ( 'NONE', #5036, .T. ) ;
#5506=CARTESIAN_POINT ( 'NONE',  ( -27.15769640663939555, -117.1457019118819005, -25.15769640663944173 ) ) ;
#5510=ORIENTED_EDGE ( 'NONE', *, *, #8446, .F. ) ;
#5513=EDGE_CURVE ( 'NONE', #1149, #4585, #9431, .T. ) ;
#5515=ORIENTED_EDGE ( 'NONE', *, *, #803, .F. ) ;
#5516=CARTESIAN_POINT ( 'NONE',  ( -50.00000000000002842, -133.6309146189979344, -23.64292728780891650 ) ) ;
#5517=CARTESIAN_POINT ( 'NONE',  ( -27.15769640663939555, -117.1457019118819005, -27.15769640663944173 ) ) ;
#5520=AXIS2_PLACEMENT_3D ( 'NONE', #2169, #8632, #583 ) ;
#5521=FACE_OUTER_BOUND ( 'NONE', #8643, .T. ) ;
#5524=DIRECTION ( 'NONE',  ( -1.000000000000000000, -0.000000000000000000, -0.000000000000000000 ) ) ;
#5525=ADVANCED_FACE ( 'NONE', ( #4825 ), #2552, .F. ) ;
#5527=EDGE_CURVE ( 'NONE', #2815, #7140, #7274, .T. ) ;
#5530=CARTESIAN_POINT ( 'NONE',  ( -27.15769640663939555, -115.1457019118818863, -23.15769640663943463 ) ) ;
#5535=FACE_OUTER_BOUND ( 'NONE', #5177, .T. ) ;
#5536=LINE ( 'NONE', #1463, #8556 ) ;
#5538=ORIENTED_EDGE ( 'NONE', *, *, #7351, .F. ) ;
#5539=CARTESIAN_POINT ( 'NONE',  ( 0.000000000000000000, -133.1457019118818721, 27.15769640663938489 ) ) ;
#5542=VERTEX_POINT ( 'NONE', #1756 ) ;
#5547=VECTOR ( 'NONE', #5995, 1000.000000000000000 ) ;
#5548=ORIENTED_EDGE ( 'NONE', *, *, #8300, .F. ) ;
#5550=DIRECTION ( 'NONE',  ( 8.379529552680124346E-16, 0.000000000000000000, -1.000000000000000000 ) ) ;
#5552=DIRECTION ( 'NONE',  ( 0.000000000000000000, 0.000000000000000000, -1.000000000000000000 ) ) ;
#5553=CARTESIAN_POINT ( 'NONE',  ( -50.00000000000001421, -145.1457019118819005, -40.00000000000002132 ) ) ;
#5554=DIRECTION ( 'NONE',  ( 0.000000000000000000, 1.000000000000000000, 0.000000000000000000 ) ) ;
#5559=CIRCLE ( 'NONE', #149, 7.525240063345735919 ) ;
#5560=ORIENTED_EDGE ( 'NONE', *, *, #6341, .F. ) ;
#5562=VECTOR ( 'NONE', #5970, 1000.000000000000000 ) ;
#5563=DIRECTION ( 'NONE',  ( 0.000000000000000000, -1.000000000000000000, 0.000000000000000000 ) ) ;
#5567=SPHERICAL_SURFACE ( 'NONE', #2450, 2.000000000000000000 ) ;
#5568=AXIS2_PLACEMENT_3D ( 'NONE', #7609, #3791, #4476 ) ;
#5569=ORIENTED_EDGE ( 'NONE', *, *, #4710, .T. ) ;
#5570=ORIENTED_EDGE ( 'NONE', *, *, #6249, .T. ) ;
#5572=CIRCLE ( 'NONE', #8960, 5.000000000000000888 ) ;
#5578=AXIS2_PLACEMENT_3D ( 'NONE', #7572, #2693, #5920 ) ;
#5579=DIRECTION ( 'NONE',  ( -1.000000000000000000, 0.000000000000000000, 0.000000000000000000 ) ) ;
#5580=EDGE_LOOP ( 'NONE', ( #1226, #3921, #1108, #10450 ) ) ;
#5587=DIRECTION ( 'NONE',  ( 0.6585271261848804070, -0.7525569905852197428, -0.000000000000000000 ) ) ;
#5589=VERTEX_POINT ( 'NONE', #909 ) ;
#5593=PLANE ( 'NONE',  #463 ) ;
#5597=EDGE_CURVE ( 'NONE', #1304, #8738, #6685, .T. ) ;
#5600=DIRECTION ( 'NONE',  ( 1.000000000000000000, 0.000000000000000000, -0.000000000000000000 ) ) ;
#5601=CARTESIAN_POINT ( 'NONE',  ( -16.29350689640809691, -115.1457019118818863, 0.000000000000000000 ) ) ;
#5604=DIRECTION ( 'NONE',  ( 0.000000000000000000, 0.000000000000000000, 1.000000000000000000 ) ) ;
#5610=VECTOR ( 'NONE', #3786, 1000.000000000000000 ) ;
#5612=CARTESIAN_POINT ( 'NONE',  ( -38.19229777560033057, 37.08684478514405214, 12.50000000000000000 ) ) ;
#5615=ORIENTED_EDGE ( 'NONE', *, *, #6086, .F. ) ;
#5617=VERTEX_POINT ( 'NONE', #5393 ) ;
#5618=CIRCLE ( 'NONE', #8836, 3.297986701801175258 ) ;
#5620=CARTESIAN_POINT ( 'NONE',  ( 24.41866285951198634, -134.3099192498708874, 49.99999999999998579 ) ) ;
#5621=CARTESIAN_POINT ( 'NONE',  ( 23.15769640663940265, -115.1457019118818863, -50.00000000000002132 ) ) ;
#5627=LINE ( 'NONE', #3404, #2185 ) ;
#5628=CIRCLE ( 'NONE', #2411, 26.75575292317714116 ) ;
#5630=VERTEX_POINT ( 'NONE', #2605 ) ;
#5636=DIRECTION ( 'NONE',  ( 1.000000000000000000, 0.000000000000000000, 0.000000000000000000 ) ) ;
#5637=AXIS2_PLACEMENT_3D ( 'NONE', #8469, #10172, #8364 ) ;
#5639=EDGE_LOOP ( 'NONE', ( #1307, #9533, #7630, #8459 ) ) ;
#5640=CARTESIAN_POINT ( 'NONE',  ( 4.856471286862176662, 145.0444252872335937, -12.49999999999999289 ) ) ;
#5644=VECTOR ( 'NONE', #2680, 1000.000000000000000 ) ;
#5646=LINE ( 'NONE', #4222, #5482 ) ;
#5648=CARTESIAN_POINT ( 'NONE',  ( -40.00000000000002842, -135.1457019118818721, 39.99999999999997868 ) ) ;
#5651=CARTESIAN_POINT ( 'NONE',  ( -27.15769640663940976, -117.1457019118819005, 23.15769640663938134 ) ) ;
#5652=ADVANCED_FACE ( 'NONE', ( #9175 ), #6995, .T. ) ;
#5655=VERTEX_POINT ( 'NONE', #4408 ) ;
#5661=CARTESIAN_POINT ( 'NONE',  ( 37.22511195853869026, -145.1457019118819005, 30.00000000000000355 ) ) ;
#5662=ORIENTED_EDGE ( 'NONE', *, *, #2486, .F. ) ;
#5667=EDGE_CURVE ( 'NONE', #3031, #6869, #4353, .T. ) ;
#5669=DIRECTION ( 'NONE',  ( 0.000000000000000000, 0.000000000000000000, 1.000000000000000000 ) ) ;
#5671=VERTEX_POINT ( 'NONE', #7590 ) ;
#5675=VECTOR ( 'NONE', #1730, 1000.000000000000000 ) ;
#5678=DIRECTION ( 'NONE',  ( 0.000000000000000000, 0.000000000000000000, -1.000000000000000000 ) ) ;
#5680=LINE ( 'NONE', #3057, #45 ) ;
#5682=CARTESIAN_POINT ( 'NONE',  ( 17.97972049165455388, 17.84145331825995484, 30.00000000000000355 ) ) ;
#5687=VECTOR ( 'NONE', #7802, 1000.000000000000000 ) ;
#5688=SHAPE_DEFINITION_REPRESENTATION ( #9597, #1081 ) ;
#5691=ORIENTED_EDGE ( 'NONE', *, *, #1787, .T. ) ;
#5693=FACE_OUTER_BOUND ( 'NONE', #10033, .T. ) ;
#5694=DIRECTION ( 'NONE',  ( 0.000000000000000000, -1.000000000000000000, 0.000000000000000000 ) ) ;
#5697=VECTOR ( 'NONE', #1988, 1000.000000000000000 ) ;
#5698=DIRECTION ( 'NONE',  ( -1.734723475976805517E-15, 1.000000000000000000, 0.000000000000000000 ) ) ;
#5699=ADVANCED_FACE ( 'NONE', ( #5886 ), #1174, .T. ) ;
#5702=CARTESIAN_POINT ( 'NONE',  ( 37.22759939293836595, -133.1457019118818721, 25.15769640663938134 ) ) ;
#5703=AXIS2_PLACEMENT_3D ( 'NONE', #9878, #6682, #1909 ) ;
#5704=ORIENTED_EDGE ( 'NONE', *, *, #1026, .F. ) ;
#5706=DIRECTION ( 'NONE',  ( -1.000000000000000000, 0.000000000000000000, 0.000000000000000000 ) ) ;
#5707=FACE_OUTER_BOUND ( 'NONE', #7136, .T. ) ;
#5709=CARTESIAN_POINT ( 'NONE',  ( -18.34874108452141783, -140.1746510883711778, -29.59847408863698703 ) ) ;
#5714=EDGE_CURVE ( 'NONE', #1670, #7639, #1812, .T. ) ;
#5716=ORIENTED_EDGE ( 'NONE', *, *, #5012, .F. ) ;
#5718=ORIENTED_EDGE ( 'NONE', *, *, #8696, .T. ) ;
#5719=DIRECTION ( 'NONE',  ( -0.000000000000000000, 1.000000000000000000, 0.000000000000000000 ) ) ;
#5720=DIRECTION ( 'NONE',  ( 0.000000000000000000, 0.000000000000000000, 1.000000000000000000 ) ) ;
#5722=DIRECTION ( 'NONE',  ( 0.000000000000000000, 0.000000000000000000, 1.000000000000000000 ) ) ;
#5723=CARTESIAN_POINT ( 'NONE',  ( -2.293506896408097795, 80.56966535057935630, -20.00000000000000711 ) ) ;
#5727=EDGE_CURVE ( 'NONE', #5912, #6555, #1065, .T. ) ;
#5729=ORIENTED_EDGE ( 'NONE', *, *, #1530, .F. ) ;
#5732=DIRECTION ( 'NONE',  ( -0.000000000000000000, -0.000000000000000000, -1.000000000000000000 ) ) ;
#5734=CARTESIAN_POINT ( 'NONE',  ( 27.15769640663937068, -133.1457019118818721, 47.99999999999997868 ) ) ;
#5735=AXIS2_PLACEMENT_3D ( 'NONE', #4908, #890, #4129 ) ;
#5736=CARTESIAN_POINT ( 'NONE',  ( 38.19229777560031636, 37.08684478514405214, 12.50000000000000000 ) ) ;
#5737=CARTESIAN_POINT ( 'NONE',  ( -2.293506896408101348, 147.5696653505793279, 30.00000000000000355 ) ) ;
#5739=ORIENTED_EDGE ( 'NONE', *, *, #803, .T. ) ;
#5743=FACE_BOUND ( 'NONE', #5029, .T. ) ;
#5744=EDGE_LOOP ( 'NONE', ( #10305, #3574, #6343, #5510 ) ) ;
#5749=CARTESIAN_POINT ( 'NONE',  ( 39.99999999999997158, -135.1457019118818721, 44.02499999999997726 ) ) ;
#5750=DIRECTION ( 'NONE',  ( -0.000000000000000000, 1.000000000000000000, -0.000000000000000000 ) ) ;
#5752=ORIENTED_EDGE ( 'NONE', *, *, #9442, .T. ) ;
#5754=ADVANCED_FACE ( 'NONE', ( #4750 ), #1578, .T. ) ;
#5755=VERTEX_POINT ( 'NONE', #2328 ) ;
#5761=CARTESIAN_POINT ( 'NONE',  ( -27.15769640663940976, -115.1457019118818863, 27.15769640663938489 ) ) ;
#5763=CONICAL_SURFACE ( 'NONE', #527, 4.025000000000000355, 0.7853981633975870569 ) ;
#5764=ORIENTED_EDGE ( 'NONE', *, *, #1961, .T. ) ;
#5765=EDGE_LOOP ( 'NONE', ( #9663, #15, #1191, #2009 ) ) ;
#5766=EDGE_LOOP ( 'NONE', ( #10071, #8819, #5718, #1123 ) ) ;
#5767=EDGE_CURVE ( 'NONE', #8114, #2357, #4346, .T. ) ;
#5768=CARTESIAN_POINT ( 'NONE',  ( 23.15769640663940265, -117.1457019118819005, -48.00000000000002132 ) ) ;
#5771=CIRCLE ( 'NONE', #9518, 10.00000000000000178 ) ;
#5774=EDGE_LOOP ( 'NONE', ( #2196, #3725, #5160, #2208 ) ) ;
#5775=CARTESIAN_POINT ( 'NONE',  ( 10.51964330236497602, 150.0000000000000000, 30.00000000000000355 ) ) ;
#5778=VECTOR ( 'NONE', #4887, 1000.000000000000000 ) ;
#5780=EDGE_LOOP ( 'NONE', ( #9142, #5341, #4895, #4971 ) ) ;
#5785=CARTESIAN_POINT ( 'NONE',  ( 73.53765631853927687, 70.39106037767953694, 30.00000000000000355 ) ) ;
#5786=EDGE_CURVE ( 'NONE', #6595, #7639, #9777, .T. ) ;
#5788=EDGE_CURVE ( 'NONE', #6846, #1518, #1534, .T. ) ;
#5790=CARTESIAN_POINT ( 'NONE',  ( -40.00000000000002842, -145.1457019118819005, 35.99999999999999289 ) ) ;
#5792=AXIS2_PLACEMENT_3D ( 'NONE', #6977, #4431, #2942 ) ;
#5793=DIRECTION ( 'NONE',  ( -1.000000000000000000, 0.000000000000000000, -6.982941293900099513E-16 ) ) ;
#5798=ORIENTED_EDGE ( 'NONE', *, *, #9423, .F. ) ;
#5799=CIRCLE ( 'NONE', #1056, 5.000000000000001776 ) ;
#5800=CARTESIAN_POINT ( 'NONE',  ( -40.00000000000001421, -135.1457019118818721, -44.02500000000001990 ) ) ;
#5801=ORIENTED_EDGE ( 'NONE', *, *, #2708, .F. ) ;
#5804=CARTESIAN_POINT ( 'NONE',  ( 14.70649310359190309, 80.56966535057935630, 16.00000000000000711 ) ) ;
#5805=DIRECTION ( 'NONE',  ( -0.000000000000000000, 1.000000000000000000, -0.000000000000000000 ) ) ;
#5809=ORIENTED_EDGE ( 'NONE', *, *, #10218, .T. ) ;
#5811=CIRCLE ( 'NONE', #4629, 7.500000000000000000 ) ;
#5812=ORIENTED_EDGE ( 'NONE', *, *, #3524, .T. ) ;
#5814=DIRECTION ( 'NONE',  ( 0.000000000000000000, 0.000000000000000000, 1.000000000000000000 ) ) ;
#5817=DIRECTION ( 'NONE',  ( 0.000000000000000000, 0.000000000000000000, 1.000000000000000000 ) ) ;
#5819=PLANE ( 'NONE',  #261 ) ;
#5827=CARTESIAN_POINT ( 'NONE',  ( -23.15769640663940976, -117.1457019118819005, 47.99999999999997868 ) ) ;
#5831=ORIENTED_EDGE ( 'NONE', *, *, #6125, .T. ) ;
#5833=EDGE_CURVE ( 'NONE', #4585, #249, #5628, .T. ) ;
#5834=CIRCLE ( 'NONE', #6520, 4.000000000000000000 ) ;
#5835=EDGE_LOOP ( 'NONE', ( #4032, #6728, #5967, #440 ) ) ;
#5837=DIRECTION ( 'NONE',  ( 0.000000000000000000, -1.000000000000000000, 0.000000000000000000 ) ) ;
#5842=CARTESIAN_POINT ( 'NONE',  ( 37.51004848672140923, -135.0890599259516875, -26.66894625761717563 ) ) ;
#5846=EDGE_CURVE ( 'NONE', #4758, #3180, #893, .T. ) ;
#5847=EDGE_CURVE ( 'NONE', #7273, #3785, #10386, .T. ) ;
#5848=ORIENTED_EDGE ( 'NONE', *, *, #10252, .T. ) ;
#5851=EDGE_LOOP ( 'NONE', ( #3853, #8103 ) ) ;
#5854=DIRECTION ( 'NONE',  ( -0.000000000000000000, 1.000000000000000000, -0.000000000000000000 ) ) ;
#5855=LINE ( 'NONE', #2524, #5675 ) ;
#5864=LINE ( 'NONE', #3276, #816 ) ;
#5866=DIRECTION ( 'NONE',  ( 0.000000000000000000, -1.000000000000000000, 0.000000000000000000 ) ) ;
#5870=CARTESIAN_POINT ( 'NONE',  ( -50.00000000000002132, -133.1457019118818721, 23.15769640663938134 ) ) ;
#5880=EDGE_CURVE ( 'NONE', #8070, #2974, #44, .T. ) ;
#5882=VECTOR ( 'NONE', #6678, 1000.000000000000000 ) ;
#5886=FACE_OUTER_BOUND ( 'NONE', #412, .T. ) ;
#5889=CIRCLE ( 'NONE', #8091, 3.999999999999996447 ) ;
#5893=CARTESIAN_POINT ( 'NONE',  ( 39.99999999999997158, -145.1457019118819005, 35.99999999999999289 ) ) ;
#5895=DIRECTION ( 'NONE',  ( 0.000000000000000000, 0.000000000000000000, 1.000000000000000000 ) ) ;
#5897=CARTESIAN_POINT ( 'NONE',  ( 37.22759939293836595, -133.2806705862436729, -25.15769640663938489 ) ) ;
#5898=ORIENTED_EDGE ( 'NONE', *, *, #9521, .T. ) ;
#5902=LINE ( 'NONE', #2675, #8444 ) ;
#5904=VECTOR ( 'NONE', #210, 1000.000000000000000 ) ;
#5912=VERTEX_POINT ( 'NONE', #3480 ) ;
#5914=ORIENTED_EDGE ( 'NONE', *, *, #6583, .F. ) ;
#5915=DIRECTION ( 'NONE',  ( -1.000000000000000000, -0.000000000000000000, -0.000000000000000000 ) ) ;
#5916=EDGE_CURVE ( 'NONE', #826, #7105, #4674, .T. ) ;
#5919=EDGE_CURVE ( 'NONE', #5357, #5066, #220, .T. ) ;
#5920=DIRECTION ( 'NONE',  ( 0.07334937666141724821, -0.9973063064792989652, 0.000000000000000000 ) ) ;
#5921=DIRECTION ( 'NONE',  ( -0.000000000000000000, 1.000000000000000000, -0.000000000000000000 ) ) ;
#5922=CARTESIAN_POINT ( 'NONE',  ( 6.756858349438879863, 146.7073643690755773, -30.00000000000000355 ) ) ;
#5924=ORIENTED_EDGE ( 'NONE', *, *, #5335, .F. ) ;
#5927=DIRECTION ( 'NONE',  ( 0.000000000000000000, 0.000000000000000000, 1.000000000000000000 ) ) ;
#5928=DIRECTION ( 'NONE',  ( 1.000000000000000000, 0.000000000000000000, 0.000000000000000000 ) ) ;
#5930=DIRECTION ( 'NONE',  ( -0.000000000000000000, -0.000000000000000000, -1.000000000000000000 ) ) ;
#5933=VERTEX_POINT ( 'NONE', #9100 ) ;
#5939=VECTOR ( 'NONE', #9075, 1000.000000000000000 ) ;
#5941=CYLINDRICAL_SURFACE ( 'NONE', #3661, 10.00000000000000178 ) ;
#5942=FACE_OUTER_BOUND ( 'NONE', #4421, .T. ) ;
#5946=VERTEX_POINT ( 'NONE', #4120 ) ;
#5947=TOROIDAL_SURFACE ( 'NONE', #9523, 4.000000000000000000, 2.000000000000000000 ) ;
#5954=AXIS2_PLACEMENT_3D ( 'NONE', #6661, #2471, #5698 ) ;
#5958=DIRECTION ( 'NONE',  ( 0.000000000000000000, 0.000000000000000000, 1.000000000000000000 ) ) ;
#5961=DIRECTION ( 'NONE',  ( 0.000000000000000000, 0.000000000000000000, 1.000000000000000000 ) ) ;
#5962=VECTOR ( 'NONE', #1599, 1000.000000000000000 ) ;
#5963=CIRCLE ( 'NONE', #3775, 1.999999999999998224 ) ;
#5964=ORIENTED_EDGE ( 'NONE', *, *, #5096, .T. ) ;
#5967=ORIENTED_EDGE ( 'NONE', *, *, #9521, .F. ) ;
#5970=DIRECTION ( 'NONE',  ( 1.396588258780021135E-16, -0.000000000000000000, 1.000000000000000000 ) ) ;
#5973=DIRECTION ( 'NONE',  ( 0.000000000000000000, 0.000000000000000000, -1.000000000000000000 ) ) ;
#5975=FACE_OUTER_BOUND ( 'NONE', #170, .T. ) ;
#5976=ORIENTED_EDGE ( 'NONE', *, *, #7327, .T. ) ;
#5977=EDGE_CURVE ( 'NONE', #2542, #1967, #3379, .T. ) ;
#5978=ORIENTED_EDGE ( 'NONE', *, *, #6039, .F. ) ;
#5983=DIRECTION ( 'NONE',  ( 0.000000000000000000, 0.000000000000000000, 1.000000000000000000 ) ) ;
#5988=CARTESIAN_POINT ( 'NONE',  ( 53.40242741783141156, 147.5696653505793279, -30.00000000000000355 ) ) ;
#5995=DIRECTION ( 'NONE',  ( 1.000000000000000000, 0.000000000000000000, 8.379529552680125332E-16 ) ) ;
#5998=DIRECTION ( 'NONE',  ( 0.000000000000000000, 0.000000000000000000, 1.000000000000000000 ) ) ;
#5999=FACE_OUTER_BOUND ( 'NONE', #3778, .T. ) ;
#6001=VERTEX_POINT ( 'NONE', #257 ) ;
#6004=EDGE_LOOP ( 'NONE', ( #9790, #10451, #6425, #5098 ) ) ;
#6006=CARTESIAN_POINT ( 'NONE',  ( -2.293506896408094242, 152.5696653505793279, 12.50000000000000000 ) ) ;
#6010=DIRECTION ( 'NONE',  ( -0.6761648913424331830, 0.7367503238654705688, 0.000000000000000000 ) ) ;
#6011=CYLINDRICAL_SURFACE ( 'NONE', #609, 3.999999999999989786 ) ;
#6013=ORIENTED_EDGE ( 'NONE', *, *, #871, .F. ) ;
#6016=ORIENTED_EDGE ( 'NONE', *, *, #8566, .T. ) ;
#6019=DIRECTION ( 'NONE',  ( 0.000000000000000000, 0.000000000000000000, 1.000000000000000000 ) ) ;
#6022=DIRECTION ( 'NONE',  ( 0.000000000000000000, 0.000000000000000000, 1.000000000000000000 ) ) ;
#6025=CARTESIAN_POINT ( 'NONE',  ( -27.15769640663939555, -117.1457019118819005, -23.15769640663944173 ) ) ;
#6026=ADVANCED_FACE ( 'NONE', ( #10213 ), #511, .T. ) ;
#6027=DIRECTION ( 'NONE',  ( -0.9973063064792990762, -0.07334937666141773394, 0.000000000000000000 ) ) ;
#6028=FACE_OUTER_BOUND ( 'NONE', #3705, .T. ) ;
#6030=VERTEX_POINT ( 'NONE', #9361 ) ;
#6031=VECTOR ( 'NONE', #3119, 1000.000000000000000 ) ;
#6033=AXIS2_PLACEMENT_3D ( 'NONE', #10459, #8223, #7326 ) ;
#6035=ORIENTED_EDGE ( 'NONE', *, *, #6379, .F. ) ;
#6036=DIRECTION ( 'NONE',  ( 0.000000000000000000, 0.000000000000000000, -1.000000000000000000 ) ) ;
#6037=CARTESIAN_POINT ( 'NONE',  ( 37.22759939293836595, -116.8755810935459181, -25.15769640663939910 ) ) ;
#6039=EDGE_CURVE ( 'NONE', #6250, #8639, #2582, .T. ) ;
#6040=CARTESIAN_POINT ( 'NONE',  ( 23.76520584195949226, -145.1457019118819005, 49.99999999999997868 ) ) ;
#6045=DIRECTION ( 'NONE',  ( 9.776117811460147207E-16, -0.000000000000000000, -1.000000000000000000 ) ) ;
#6046=AXIS2_PLACEMENT_3D ( 'NONE', #2129, #2870, #8438 ) ;
#6049=CARTESIAN_POINT ( 'NONE',  ( -2.293506896408097795, 152.5696653505793279, 12.50000000000000000 ) ) ;
#6051=DIRECTION ( 'NONE',  ( -1.000000000000000000, -0.000000000000000000, -0.000000000000000000 ) ) ;
#6052=DIRECTION ( 'NONE',  ( 0.6585271261848795188, -0.7525569905852207420, -2.609853011491003364E-16 ) ) ;
#6057=AXIS2_PLACEMENT_3D ( 'NONE', #4403, #7632, #6036 ) ;
#6063=EDGE_CURVE ( 'NONE', #9794, #4419, #5456, .T. ) ;
#6064=LINE ( 'NONE', #8403, #6547 ) ;
#6066=CARTESIAN_POINT ( 'NONE',  ( 37.65642917125824596, -135.1457019118819005, 27.03600932663011847 ) ) ;
#6073=DIRECTION ( 'NONE',  ( 0.6585271261848804070, -0.7525569905852197428, -0.000000000000000000 ) ) ;
#6077=LINE ( 'NONE', #2898, #5562 ) ;
#6078=PLANE ( 'NONE',  #6806 ) ;
#6079=VERTEX_POINT ( 'NONE', #8561 ) ;
#6080=CARTESIAN_POINT ( 'NONE',  ( -40.00000000000002842, -145.1457019118819005, 39.99999999999997868 ) ) ;
#6081=CARTESIAN_POINT ( 'NONE',  ( -48.00000000000002132, -133.1457019118818721, 23.15769640663938134 ) ) ;
#6084=VECTOR ( 'NONE', #8484, 1000.000000000000000 ) ;
#6086=EDGE_CURVE ( 'NONE', #6250, #6120, #2890, .T. ) ;
#6088=CARTESIAN_POINT ( 'NONE',  ( 4.856471286862175774, 152.5696653505793279, 25.00000000000000000 ) ) ;
#6090=DIRECTION ( 'NONE',  ( -1.000000000000000000, 0.000000000000000000, 0.000000000000000000 ) ) ;
#6092=DIRECTION ( 'NONE',  ( -0.000000000000000000, 1.000000000000000000, -0.000000000000000000 ) ) ;
#6094=VERTEX_POINT ( 'NONE', #8511 ) ;
#6095=ORIENTED_EDGE ( 'NONE', *, *, #4375, .T. ) ;
#6096=EDGE_CURVE ( 'NONE', #2136, #847, #8458, .T. ) ;
#6098=ORIENTED_EDGE ( 'NONE', *, *, #7309, .F. ) ;
#6099=CARTESIAN_POINT ( 'NONE',  ( 27.15769640663940621, -135.1457019118818721, -48.00000000000002132 ) ) ;
#6102=CARTESIAN_POINT ( 'NONE',  ( -2.293506896408097795, 37.08684478514406635, 30.00000000000000355 ) ) ;
#6104=DIRECTION ( 'NONE',  ( 0.000000000000000000, -1.000000000000000000, 0.000000000000000000 ) ) ;
#6105=ORIENTED_EDGE ( 'NONE', *, *, #3968, .T. ) ;
#6108=ADVANCED_FACE ( 'NONE', ( #9256 ), #4537, .T. ) ;
#6109=ADVANCED_FACE ( 'NONE', ( #1887 ), #8332, .T. ) ;
#6112=PLANE ( 'NONE',  #8076 ) ;
#6119=EDGE_CURVE ( 'NONE', #7774, #5230, #1094, .T. ) ;
#6120=VERTEX_POINT ( 'NONE', #6765 ) ;
#6124=AXIS2_PLACEMENT_3D ( 'NONE', #919, #2561, #1713 ) ;
#6125=EDGE_CURVE ( 'NONE', #9884, #4360, #5618, .T. ) ;
#6126=LINE ( 'NONE', #2098, #1642 ) ;
#6128=ORIENTED_EDGE ( 'NONE', *, *, #7942, .F. ) ;
#6130=CARTESIAN_POINT ( 'NONE',  ( -20.14472382240651882, -141.8229441850657793, 28.16739522765904624 ) ) ;
#6131=DIRECTION ( 'NONE',  ( 0.000000000000000000, -1.000000000000000000, -0.000000000000000000 ) ) ;
#6133=CARTESIAN_POINT ( 'NONE',  ( -40.00000000000001421, -135.1457019118818721, -50.00000000000002132 ) ) ;
#6136=CIRCLE ( 'NONE', #1567, 2.000000000000001776 ) ;
#6138=AXIS2_PLACEMENT_3D ( 'NONE', #7285, #1720, #867 ) ;
#6139=ORIENTED_EDGE ( 'NONE', *, *, #6324, .F. ) ;
#6141=VECTOR ( 'NONE', #5930, 1000.000000000000000 ) ;
#6142=ORIENTED_EDGE ( 'NONE', *, *, #4004, .F. ) ;
#6144=DIRECTION ( 'NONE',  ( -1.000000000000000000, 0.000000000000000000, 0.000000000000000000 ) ) ;
#6145=CYLINDRICAL_SURFACE ( 'NONE', #3615, 4.000000000000000000 ) ;
#6147=CARTESIAN_POINT ( 'NONE',  ( 42.22511195853867605, 17.84145331825995839, 25.00000000000000000 ) ) ;
#6149=ORIENTED_EDGE ( 'NONE', *, *, #7351, .T. ) ;
#6150=AXIS2_PLACEMENT_3D ( 'NONE', #6025, #9269, #1209 ) ;
#6152=ORIENTED_EDGE ( 'NONE', *, *, #7944, .T. ) ;
#6154=CARTESIAN_POINT ( 'NONE',  ( 94.78677303995212355, -145.1457019118819005, 30.00000000000000355 ) ) ;
#6157=DIRECTION ( 'NONE',  ( 0.000000000000000000, 1.000000000000000000, 0.000000000000000000 ) ) ;
#6160=DIRECTION ( 'NONE',  ( 0.000000000000000000, 0.000000000000000000, -1.000000000000000000 ) ) ;
#6165=CARTESIAN_POINT ( 'NONE',  ( 37.71464122736490054, -135.1457019118818721, -27.15769640663940265 ) ) ;
#6167=LINE ( 'NONE', #5426, #806 ) ;
#6168=DIRECTION ( 'NONE',  ( 1.000000000000000000, 0.000000000000000000, 1.734723475976805517E-15 ) ) ;
#6169=EDGE_CURVE ( 'NONE', #7935, #8658, #882, .T. ) ;
#6170=DIRECTION ( 'NONE',  ( -0.000000000000000000, 1.000000000000000000, -0.000000000000000000 ) ) ;
#6171=ADVANCED_FACE ( 'NONE', ( #4584 ), #9527, .F. ) ;
#6172=ORIENTED_EDGE ( 'NONE', *, *, #7289, .F. ) ;
#6173=DIRECTION ( 'NONE',  ( -0.000000000000000000, 1.000000000000000000, 0.000000000000000000 ) ) ;
#6177=CARTESIAN_POINT ( 'NONE',  ( 10.51964330236497602, 150.0000000000000000, 30.00000000000000355 ) ) ;
#6178=ORIENTED_EDGE ( 'NONE', *, *, #6096, .T. ) ;
#6179=AXIS2_PLACEMENT_3D ( 'NONE', #9159, #2053, #3755 ) ;
#6182=FACE_OUTER_BOUND ( 'NONE', #3536, .T. ) ;
#6183=ORIENTED_EDGE ( 'NONE', *, *, #8765, .T. ) ;
#6184=DIRECTION ( 'NONE',  ( 0.000000000000000000, 0.000000000000000000, 1.000000000000000000 ) ) ;
#6185=CARTESIAN_POINT ( 'NONE',  ( 4.856471286862173997, 152.5696653505793279, -12.50000000000000000 ) ) ;
#6186=EDGE_CURVE ( 'NONE', #4407, #2391, #5431, .T. ) ;
#6187=ADVANCED_FACE ( 'NONE', ( #3049 ), #3956, .F. ) ;
#6191=DIRECTION ( 'NONE',  ( 0.000000000000000000, 0.000000000000000000, 1.000000000000000000 ) ) ;
#6193=ORIENTED_EDGE ( 'NONE', *, *, #1961, .F. ) ;
#6194=CYLINDRICAL_SURFACE ( 'NONE', #5520, 2.000000000000001776 ) ;
#6197=FACE_OUTER_BOUND ( 'NONE', #8710, .T. ) ;
#6198=CONICAL_SURFACE ( 'NONE', #9071, 4.025000000000000355, 0.7853981633975870569 ) ;
#6200=CARTESIAN_POINT ( 'NONE',  ( -50.00000000000002132, -134.8487249201535008, 25.28852788137215057 ) ) ;
#6203=LINE ( 'NONE', #2179, #5498 ) ;
#6208=ADVANCED_FACE ( 'NONE', ( #7187 ), #8616, .F. ) ;
#6209=ORIENTED_EDGE ( 'NONE', *, *, #142, .T. ) ;
#6210=ORIENTED_EDGE ( 'NONE', *, *, #8699, .T. ) ;
#6212=CARTESIAN_POINT ( 'NONE',  ( 25.93998375192765948, -135.0799149511624364, 49.99999999999997868 ) ) ;
#6214=LINE ( 'NONE', #1286, #9942 ) ;
#6215=CARTESIAN_POINT ( 'NONE',  ( -27.15769640663939555, -133.1457019118818721, -27.15769640663944173 ) ) ;
#6217=LINE ( 'NONE', #1398, #6884 ) ;
#6218=ORIENTED_EDGE ( 'NONE', *, *, #5008, .F. ) ;
#6221=ORIENTED_EDGE ( 'NONE', *, *, #6575, .F. ) ;
#6223=CARTESIAN_POINT ( 'NONE',  ( 49.99999999999997158, -135.1457019118818721, 39.99999999999997868 ) ) ;
#6225=DIRECTION ( 'NONE',  ( -0.000000000000000000, 1.000000000000000000, -0.000000000000000000 ) ) ;
#6227=ORIENTED_EDGE ( 'NONE', *, *, #6481, .F. ) ;
#6228=CARTESIAN_POINT ( 'NONE',  ( 27.15769640663936357, -133.1457019118818721, -3.792811993702490094E-15 ) ) ;
#6229=ORIENTED_EDGE ( 'NONE', *, *, #6850, .T. ) ;
#6232=CIRCLE ( 'NONE', #8770, 2.000000000000001776 ) ;
#6234=EDGE_CURVE ( 'NONE', #3054, #3508, #6645, .T. ) ;
#6236=ORIENTED_EDGE ( 'NONE', *, *, #9064, .T. ) ;
#6239=ORIENTED_EDGE ( 'NONE', *, *, #2427, .F. ) ;
#6240=DIRECTION ( 'NONE',  ( 0.000000000000000000, 0.000000000000000000, 1.000000000000000000 ) ) ;
#6243=DIRECTION ( 'NONE',  ( 0.000000000000000000, 0.000000000000000000, 1.000000000000000000 ) ) ;
#6246=LINE ( 'NONE', #637, #7727 ) ;
#6249=EDGE_CURVE ( 'NONE', #869, #7130, #2313, .T. ) ;
#6250=VERTEX_POINT ( 'NONE', #3153 ) ;
#6251=CARTESIAN_POINT ( 'NONE',  ( 27.15769640663938489, -115.1457019118818863, -27.15769640663940976 ) ) ;
#6252=FACE_BOUND ( 'NONE', #9600, .T. ) ;
#6254=ORIENTED_EDGE ( 'NONE', *, *, #1904, .T. ) ;
#6256=DIRECTION ( 'NONE',  ( 1.000000000000000000, 0.000000000000000000, 0.000000000000000000 ) ) ;
#6257=FACE_OUTER_BOUND ( 'NONE', #7145, .T. ) ;
#6261=VERTEX_POINT ( 'NONE', #717 ) ;
#6263=ADVANCED_FACE ( 'NONE', ( #4006 ), #1401, .F. ) ;
#6264=ORIENTED_EDGE ( 'NONE', *, *, #9305, .T. ) ;
#6266=LINE ( 'NONE', #3395, #3759 ) ;
#6267=DIRECTION ( 'NONE',  ( -0.000000000000000000, 1.000000000000000000, -0.000000000000000000 ) ) ;
#6269=PLANE ( 'NONE',  #7900 ) ;
#6270=VERTEX_POINT ( 'NONE', #8666 ) ;
#6271=CARTESIAN_POINT ( 'NONE',  ( 2.275687196221499263E-14, -135.1457019118818721, -27.15769640663943107 ) ) ;
#6273=LINE ( 'NONE', #6478, #4527 ) ;
#6276=EDGE_CURVE ( 'NONE', #4046, #8070, #1382, .T. ) ;
#6277=DIRECTION ( 'NONE',  ( 0.000000000000000000, 1.000000000000000000, 0.000000000000000000 ) ) ;
#6278=ORIENTED_EDGE ( 'NONE', *, *, #5513, .F. ) ;
#6280=CARTESIAN_POINT ( 'NONE',  ( -40.00000000000001421, -145.1457019118819005, -40.00000000000002132 ) ) ;
#6281=ORIENTED_EDGE ( 'NONE', *, *, #3140, .F. ) ;
#6286=ORIENTED_EDGE ( 'NONE', *, *, #5597, .T. ) ;
#6290=LINE ( 'NONE', #3964, #1429 ) ;
#6292=CARTESIAN_POINT ( 'NONE',  ( 4.856471286862176662, 145.0444252872335937, 25.00000000000000000 ) ) ;
#6294=EDGE_CURVE ( 'NONE', #7113, #7523, #977, .T. ) ;
#6295=CIRCLE ( 'NONE', #3073, 2.000000000000001776 ) ;
#6297=ORIENTED_EDGE ( 'NONE', *, *, #2280, .F. ) ;
#6299=ORIENTED_EDGE ( 'NONE', *, *, #1188, .F. ) ;
#6302=AXIS2_PLACEMENT_3D ( 'NONE', #7829, #573, #3808 ) ;
#6304=AXIS2_PLACEMENT_3D ( 'NONE', #7563, #1197, #5269 ) ;
#6306=DIRECTION ( 'NONE',  ( -1.000000000000000000, -0.000000000000000000, -0.000000000000000000 ) ) ;
#6307=DIRECTION ( 'NONE',  ( 0.000000000000000000, 0.000000000000000000, -1.000000000000000000 ) ) ;
#6308=EDGE_LOOP ( 'NONE', ( #1674, #7212, #3256, #10139 ) ) ;
#6309=EDGE_CURVE ( 'NONE', #3675, #4386, #9682, .T. ) ;
#6310=EDGE_CURVE ( 'NONE', #6574, #9459, #2622, .T. ) ;
#6312=ORIENTED_EDGE ( 'NONE', *, *, #1643, .T. ) ;
#6313=AXIS2_PLACEMENT_3D ( 'NONE', #6215, #3569, #5998 ) ;
#6316=VERTEX_POINT ( 'NONE', #3417 ) ;
#6317=CARTESIAN_POINT ( 'NONE',  ( 0.000000000000000000, -135.1457019118818721, 0.000000000000000000 ) ) ;
#6318=DIRECTION ( 'NONE',  ( 0.000000000000000000, -1.000000000000000000, 0.000000000000000000 ) ) ;
#6320=CARTESIAN_POINT ( 'NONE',  ( 0.000000000000000000, -145.1457019118819005, 49.99999999999997868 ) ) ;
#6323=DIRECTION ( 'NONE',  ( -0.000000000000000000, 1.000000000000000000, -0.000000000000000000 ) ) ;
#6324=EDGE_CURVE ( 'NONE', #1005, #9303, #9791, .T. ) ;
#6326=ORIENTED_EDGE ( 'NONE', *, *, #3849, .F. ) ;
#6327=FACE_OUTER_BOUND ( 'NONE', #9846, .T. ) ;
#6335=EDGE_LOOP ( 'NONE', ( #9194, #3458, #1965, #4568, #7253, #3901 ) ) ;
#6341=EDGE_CURVE ( 'NONE', #7279, #1670, #10208, .T. ) ;
#6343=ORIENTED_EDGE ( 'NONE', *, *, #9653, .F. ) ;
#6344=CARTESIAN_POINT ( 'NONE',  ( -18.34874108452141783, -140.1746510883711778, 24.43989726270226370 ) ) ;
#6348=FACE_OUTER_BOUND ( 'NONE', #7524, .T. ) ;
#6350=AXIS2_PLACEMENT_3D ( 'NONE', #1589, #694, #6307 ) ;
#6351=ORIENTED_EDGE ( 'NONE', *, *, #5786, .T. ) ;
#6352=DIRECTION ( 'NONE',  ( 0.000000000000000000, 1.000000000000000000, 0.000000000000000000 ) ) ;
#6353=ORIENTED_EDGE ( 'NONE', *, *, #2945, .F. ) ;
#6364=CIRCLE ( 'NONE', #3839, 3.297986701801175258 ) ;
#6368=LINE ( 'NONE', #8807, #4436 ) ;
#6370=CARTESIAN_POINT ( 'NONE',  ( -50.00000000000002132, -117.1457019118819005, -23.15769640663945594 ) ) ;
#6372=AXIS2_PLACEMENT_3D ( 'NONE', #3757, #1963, #335 ) ;
#6373=VERTEX_POINT ( 'NONE', #8182 ) ;
#6377=EDGE_CURVE ( 'NONE', #2339, #86, #8238, .T. ) ;
#6378=DIRECTION ( 'NONE',  ( 1.000000000000000000, 0.000000000000000000, 9.776117811460135374E-16 ) ) ;
#6379=EDGE_CURVE ( 'NONE', #541, #10221, #6994, .T. ) ;
#6380=ADVANCED_FACE ( 'NONE', ( #7391 ), #8984, .F. ) ;
#6381=CARTESIAN_POINT ( 'NONE',  ( 23.40006363390417832, -133.3880685335015812, -50.00000000000001421 ) ) ;
#6383=CIRCLE ( 'NONE', #10116, 2.000000000000001776 ) ;
#6384=ORIENTED_EDGE ( 'NONE', *, *, #1846, .F. ) ;
#6388=ORIENTED_EDGE ( 'NONE', *, *, #1656, .T. ) ;
#6389=CARTESIAN_POINT ( 'NONE',  ( -23.15769640663937423, -117.1457019118819005, -48.00000000000002132 ) ) ;
#6391=VECTOR ( 'NONE', #2384, 1000.000000000000000 ) ;
#6392=ADVANCED_FACE ( 'NONE', ( #8128 ), #5053, .F. ) ;
#6393=ORIENTED_EDGE ( 'NONE', *, *, #933, .T. ) ;
#6395=FACE_OUTER_BOUND ( 'NONE', #10276, .T. ) ;
#6398=CIRCLE ( 'NONE', #4033, 3.297986701801175258 ) ;
#6401=CIRCLE ( 'NONE', #8268, 3.297986701801175258 ) ;
#6407=DIRECTION ( 'NONE',  ( 0.000000000000000000, 0.000000000000000000, 1.000000000000000000 ) ) ;
#6408=CARTESIAN_POINT ( 'NONE',  ( -23.15769640663940976, -117.1457019118819005, -1.617088345095243827E-14 ) ) ;
#6410=ORIENTED_EDGE ( 'NONE', *, *, #5332, .F. ) ;
#6411=ADVANCED_FACE ( 'NONE', ( #1029 ), #6485, .T. ) ;
#6412=EDGE_LOOP ( 'NONE', ( #8400, #178, #6906, #6684, #813, #1602, #6476, #7897, #8568, #8213, #8609, #8327, #7367, #5848 ) ) ;
#6415=FACE_OUTER_BOUND ( 'NONE', #1747, .T. ) ;
#6419=DIRECTION ( 'NONE',  ( -0.000000000000000000, -0.000000000000000000, -1.000000000000000000 ) ) ;
#6420=ORIENTED_EDGE ( 'NONE', *, *, #2088, .T. ) ;
#6424=ORIENTED_EDGE ( 'NONE', *, *, #554, .T. ) ;
#6425=ORIENTED_EDGE ( 'NONE', *, *, #1306, .T. ) ;
#6426=DIRECTION ( 'NONE',  ( 0.000000000000000000, 0.000000000000000000, 1.000000000000000000 ) ) ;
#6427=LINE ( 'NONE', #5736, #3633 ) ;
#6429=CARTESIAN_POINT ( 'NONE',  ( -16.29350689640809691, -140.1746510883711778, -27.01918567566963247 ) ) ;
#6430=EDGE_LOOP ( 'NONE', ( #3701, #7717, #8540 ) ) ;
#6431=CARTESIAN_POINT ( 'NONE',  ( -2.293506896408097795, 42.08684478514406635, -25.00000000000000355 ) ) ;
#6435=ORIENTED_EDGE ( 'NONE', *, *, #4035, .T. ) ;
#6439=FACE_OUTER_BOUND ( 'NONE', #9587, .T. ) ;
#6440=AXIS2_PLACEMENT_3D ( 'NONE', #4273, #3479, #4169 ) ;
#6442=CARTESIAN_POINT ( 'NONE',  ( -26.62179802177712773, -135.1457019118818721, -50.00000000000002132 ) ) ;
#6444=DIRECTION ( 'NONE',  ( -0.000000000000000000, 1.000000000000000000, -0.000000000000000000 ) ) ;
#6447=EDGE_CURVE ( 'NONE', #7344, #1239, #6474, .T. ) ;
#6449=CIRCLE ( 'NONE', #8141, 2.000000000000001776 ) ;
#6450=CARTESIAN_POINT ( 'NONE',  ( 39.99999999999997158, -135.1457019118818721, 49.99999999999997868 ) ) ;
#6452=ORIENTED_EDGE ( 'NONE', *, *, #6377, .T. ) ;
#6453=DIRECTION ( 'NONE',  ( -1.000000000000000000, -0.000000000000000000, -0.000000000000000000 ) ) ;
#6454=DIRECTION ( 'NONE',  ( 0.000000000000000000, 0.000000000000000000, 1.000000000000000000 ) ) ;
#6457=CARTESIAN_POINT ( 'NONE',  ( -40.00000000000002842, -145.1457019118819005, 39.99999999999997868 ) ) ;
#6462=VERTEX_POINT ( 'NONE', #1187 ) ;
#6468=CARTESIAN_POINT ( 'NONE',  ( -40.00000000000001421, -135.1457019118818721, -40.00000000000002132 ) ) ;
#6471=CARTESIAN_POINT ( 'NONE',  ( 0.000000000000000000, -115.1457019118818863, 25.15769640663938134 ) ) ;
#6474=CIRCLE ( 'NONE', #3608, 4.000000000000000000 ) ;
#6475=LINE ( 'NONE', #127, #8955 ) ;
#6476=ORIENTED_EDGE ( 'NONE', *, *, #8123, .F. ) ;
#6478=CARTESIAN_POINT ( 'NONE',  ( -50.00000000000002132, -135.1457019118818721, -6.938893903907231533E-15 ) ) ;
#6479=AXIS2_PLACEMENT_3D ( 'NONE', #174, #1699, #1752 ) ;
#6481=EDGE_CURVE ( 'NONE', #3054, #7273, #3685, .T. ) ;
#6485=CYLINDRICAL_SURFACE ( 'NONE', #5437, 5.000000000000000888 ) ;
#6487=EDGE_LOOP ( 'NONE', ( #3275, #3528, #425, #1214 ) ) ;
#6488=CIRCLE ( 'NONE', #9204, 5.000000000000000888 ) ;
#6492=( BOUNDED_CURVE ( )  B_SPLINE_CURVE ( 3, ( #3987, #1447, #7219, #8858 ),
 .UNSPECIFIED., .F., .T. ) 
 B_SPLINE_CURVE_WITH_KNOTS ( ( 4, 4 ),
 ( 2.243596561310088777, 4.039588745869492570 ),
 .UNSPECIFIED. ) 
 CURVE ( )  GEOMETRIC_REPRESENTATION_ITEM ( )  RATIONAL_B_SPLINE_CURVE ( ( 1.000000000000000000, 0.7487856226529291392, 0.7487856226529291392, 1.000000000000000000 ) ) 
 REPRESENTATION_ITEM ( '' )  );
#6495=CARTESIAN_POINT ( 'NONE',  ( 4.856471286862176662, 145.0444252872335937, 30.00000000000000355 ) ) ;
#6497=CIRCLE ( 'NONE', #5314, 4.999999999999995559 ) ;
#6500=ORIENTED_EDGE ( 'NONE', *, *, #7804, .F. ) ;
#6501=CIRCLE ( 'NONE', #1087, 10.00000000000000178 ) ;
#6504=ORIENTED_EDGE ( 'NONE', *, *, #5335, .T. ) ;
#6505=CARTESIAN_POINT ( 'NONE',  ( -40.00000000000001421, -135.1707019118818778, -36.00000000000002842 ) ) ;
#6508=EDGE_CURVE ( 'NONE', #7051, #3749, #7652, .T. ) ;
#6509=EDGE_CURVE ( 'NONE', #9955, #9452, #9998, .T. ) ;
#6513=FACE_OUTER_BOUND ( 'NONE', #8515, .T. ) ;
#6515=ORIENTED_EDGE ( 'NONE', *, *, #9660, .T. ) ;
#6516=AXIS2_PLACEMENT_3D ( 'NONE', #8897, #5023, #269 ) ;
#6518=ORIENTED_EDGE ( 'NONE', *, *, #9035, .F. ) ;
#6519=DIRECTION ( 'NONE',  ( -1.000000000000000000, 0.000000000000000000, 0.000000000000000000 ) ) ;
#6520=AXIS2_PLACEMENT_3D ( 'NONE', #7888, #629, #3869 ) ;
#6531=VERTEX_POINT ( 'NONE', #2673 ) ;
#6533=ORIENTED_EDGE ( 'NONE', *, *, #6835, .F. ) ;
#6536=DIRECTION ( 'NONE',  ( -0.000000000000000000, 1.000000000000000000, -0.000000000000000000 ) ) ;
#6537=DIRECTION ( 'NONE',  ( -0.6585271261848804070, 0.7525569905852197428, -0.000000000000000000 ) ) ;
#6538=VECTOR ( 'NONE', #25, 1000.000000000000000 ) ;
#6541=ORIENTED_EDGE ( 'NONE', *, *, #1915, .F. ) ;
#6543=EDGE_CURVE ( 'NONE', #1670, #2698, #6449, .T. ) ;
#6545=ORIENTED_EDGE ( 'NONE', *, *, #6886, .T. ) ;
#6547=VECTOR ( 'NONE', #3692, 1000.000000000000000 ) ;
#6549=DIRECTION ( 'NONE',  ( 0.000000000000000000, 1.000000000000000000, 0.000000000000000000 ) ) ;
#6551=CARTESIAN_POINT ( 'NONE',  ( 37.59878849545336976, 32.08684478514406635, -12.49999999999999289 ) ) ;
#6552=DIRECTION ( 'NONE',  ( 0.000000000000000000, 0.000000000000000000, 1.000000000000000000 ) ) ;
#6555=VERTEX_POINT ( 'NONE', #9193 ) ;
#6558=ORIENTED_EDGE ( 'NONE', *, *, #8580, .F. ) ;
#6566=DIRECTION ( 'NONE',  ( -1.000000000000000000, -0.000000000000000000, -0.000000000000000000 ) ) ;
#6567=CYLINDRICAL_SURFACE ( 'NONE', #92, 2.000000000000001776 ) ;
#6571=ORIENTED_EDGE ( 'NONE', *, *, #2033, .T. ) ;
#6572=EDGE_CURVE ( 'NONE', #7421, #7191, #5464, .T. ) ;
#6574=VERTEX_POINT ( 'NONE', #1875 ) ;
#6575=EDGE_CURVE ( 'NONE', #3699, #4400, #8169, .T. ) ;
#6576=AXIS2_PLACEMENT_3D ( 'NONE', #6251, #2281, #7157 ) ;
#6580=CARTESIAN_POINT ( 'NONE',  ( 37.59878849545336976, 32.08684478514406635, 12.50000000000000355 ) ) ;
#6583=EDGE_CURVE ( 'NONE', #5111, #6849, #5963, .T. ) ;
#6588=AXIS2_PLACEMENT_3D ( 'NONE', #4162, #144, #8292 ) ;
#6589=ORIENTED_EDGE ( 'NONE', *, *, #9365, .F. ) ;
#6592=CIRCLE ( 'NONE', #2021, 3.999999999999989786 ) ;
#6593=FACE_OUTER_BOUND ( 'NONE', #5835, .T. ) ;
#6595=VERTEX_POINT ( 'NONE', #552 ) ;
#6598=EDGE_LOOP ( 'NONE', ( #4190, #6515, #7595, #9899 ) ) ;
#6599=DIRECTION ( 'NONE',  ( 0.000000000000000000, 0.000000000000000000, 1.000000000000000000 ) ) ;
#6600=VERTEX_POINT ( 'NONE', #2932 ) ;
#6602=EDGE_LOOP ( 'NONE', ( #9036, #2759 ) ) ;
#6603=EDGE_CURVE ( 'NONE', #4826, #7421, #8708, .T. ) ;
#6604=CARTESIAN_POINT ( 'NONE',  ( -48.00000000000002132, -115.1457019118818863, -25.15769640663945950 ) ) ;
#6605=CARTESIAN_POINT ( 'NONE',  ( -2.293506896408101348, 42.08684478514406635, 25.00000000000000000 ) ) ;
#6606=DIRECTION ( 'NONE',  ( -1.000000000000000000, 0.000000000000000000, 0.000000000000000000 ) ) ;
#6610=ORIENTED_EDGE ( 'NONE', *, *, #9035, .T. ) ;
#6611=DIRECTION ( 'NONE',  ( -0.000000000000000000, 1.000000000000000000, -0.000000000000000000 ) ) ;
#6612=CYLINDRICAL_SURFACE ( 'NONE', #204, 5.000000000000000888 ) ;
#6614=DIRECTION ( 'NONE',  ( 0.000000000000000000, 1.000000000000000000, 0.000000000000000000 ) ) ;
#6616=CYLINDRICAL_SURFACE ( 'NONE', #2788, 2.000000000000001776 ) ;
#6617=CARTESIAN_POINT ( 'NONE',  ( 27.15769640663938489, -133.1457019118818721, -27.15769640663940621 ) ) ;
#6620=EDGE_LOOP ( 'NONE', ( #3542, #6518 ) ) ;
#6621=ORIENTED_EDGE ( 'NONE', *, *, #4285, .T. ) ;
#6631=ORIENTED_EDGE ( 'NONE', *, *, #7347, .F. ) ;
#6633=ORIENTED_EDGE ( 'NONE', *, *, #9769, .T. ) ;
#6634=AXIS2_PLACEMENT_3D ( 'NONE', #5734, #7441, #9839 ) ;
#6640=CARTESIAN_POINT ( 'NONE',  ( -23.15769640663937423, -115.1457019118818863, -48.00000000000002132 ) ) ;
#6641=CARTESIAN_POINT ( 'NONE',  ( -25.15769640663940976, -115.1457019118818863, 47.99999999999997868 ) ) ;
#6643=CIRCLE ( 'NONE', #7834, 2.000000000000001776 ) ;
#6644=EDGE_CURVE ( 'NONE', #4565, #36, #2137, .T. ) ;
#6645=CIRCLE ( 'NONE', #5115, 3.999999999999996447 ) ;
#6649=CARTESIAN_POINT ( 'NONE',  ( 49.99999999999998579, -135.1457019118818721, -40.00000000000002132 ) ) ;
#6653=DIRECTION ( 'NONE',  ( 0.000000000000000000, 0.000000000000000000, 1.000000000000000000 ) ) ;
#6657=CARTESIAN_POINT ( 'NONE',  ( 0.000000000000000000, -135.1457019118818721, 0.000000000000000000 ) ) ;
#6658=FACE_OUTER_BOUND ( 'NONE', #10306, .T. ) ;
#6659=AXIS2_PLACEMENT_3D ( 'NONE', #2694, #5921, #9323 ) ;
#6661=CARTESIAN_POINT ( 'NONE',  ( 23.15769640663940265, -117.1457019118819005, -48.00000000000002132 ) ) ;
#6665=AXIS2_PLACEMENT_3D ( 'NONE', #9592, #10278, #2323 ) ;
#6666=ORIENTED_EDGE ( 'NONE', *, *, #6572, .F. ) ;
#6671=FACE_OUTER_BOUND ( 'NONE', #4248, .T. ) ;
#6675=ORIENTED_EDGE ( 'NONE', *, *, #9151, .F. ) ;
#6676=VECTOR ( 'NONE', #730, 1000.000000000000000 ) ;
#6677=ORIENTED_EDGE ( 'NONE', *, *, #8525, .F. ) ;
#6678=DIRECTION ( 'NONE',  ( 1.000000000000000000, -0.000000000000000000, 0.000000000000000000 ) ) ;
#6679=CARTESIAN_POINT ( 'NONE',  ( -2.293506896408097795, 152.5696653505793279, 25.00000000000000000 ) ) ;
#6682=DIRECTION ( 'NONE',  ( -0.000000000000000000, 1.000000000000000000, -0.000000000000000000 ) ) ;
#6683=AXIS2_PLACEMENT_3D ( 'NONE', #9661, #7262, #6407 ) ;
#6684=ORIENTED_EDGE ( 'NONE', *, *, #4779, .T. ) ;
#6685=LINE ( 'NONE', #9986, #5187 ) ;
#6686=ORIENTED_EDGE ( 'NONE', *, *, #6249, .F. ) ;
#6687=ADVANCED_FACE ( 'NONE', ( #6327 ), #9572, .F. ) ;
#6690=LINE ( 'NONE', #1664, #5939 ) ;
#6691=CYLINDRICAL_SURFACE ( 'NONE', #944, 3.999999999999989786 ) ;
#6692=DIRECTION ( 'NONE',  ( -0.000000000000000000, -0.000000000000000000, -1.000000000000000000 ) ) ;
#6695=AXIS2_PLACEMENT_3D ( 'NONE', #6867, #6761, #1299 ) ;
#6699=VERTEX_POINT ( 'NONE', #9460 ) ;
#6704=ORIENTED_EDGE ( 'NONE', *, *, #46, .T. ) ;
#6705=CIRCLE ( 'NONE', #2985, 4.025000000000000355 ) ;
#6708=FACE_OUTER_BOUND ( 'NONE', #5765, .T. ) ;
#6711=CARTESIAN_POINT ( 'NONE',  ( 39.99999999999998579, -135.1457019118818721, -35.97500000000002274 ) ) ;
#6714=ORIENTED_EDGE ( 'NONE', *, *, #9660, .F. ) ;
#6715=EDGE_CURVE ( 'NONE', #3675, #2182, #5447, .T. ) ;
#6716=CARTESIAN_POINT ( 'NONE',  ( 42.22511195853868315, -135.1457019118818721, 30.00000000000000355 ) ) ;
#6719=CARTESIAN_POINT ( 'NONE',  ( 17.97972049165455388, 17.84145331825995484, -25.00000000000000355 ) ) ;
#6720=DIRECTION ( 'NONE',  ( 0.000000000000000000, 0.000000000000000000, 1.000000000000000000 ) ) ;
#6723=CARTESIAN_POINT ( 'NONE',  ( -40.00000000000002842, -135.1707019118818778, 39.99999999999997868 ) ) ;
#6726=ORIENTED_EDGE ( 'NONE', *, *, #3658, .F. ) ;
#6728=ORIENTED_EDGE ( 'NONE', *, *, #2161, .F. ) ;
#6729=DIRECTION ( 'NONE',  ( 0.000000000000000000, 0.000000000000000000, 1.000000000000000000 ) ) ;
#6735=EDGE_CURVE ( 'NONE', #1811, #2339, #1725, .T. ) ;
#6746=CARTESIAN_POINT ( 'NONE',  ( 73.53765631853929108, 70.39106037767955115, -25.00000000000000355 ) ) ;
#6749=DIRECTION ( 'NONE',  ( 0.000000000000000000, 0.000000000000000000, 1.000000000000000000 ) ) ;
#6754=CARTESIAN_POINT ( 'NONE',  ( -50.00000000000002842, -115.1457019118818863, 39.99999999999997868 ) ) ;
#6755=EDGE_LOOP ( 'NONE', ( #5739, #2123, #4041, #4493 ) ) ;
#6759=EDGE_CURVE ( 'NONE', #2974, #3710, #707, .T. ) ;
#6760=EDGE_CURVE ( 'NONE', #2186, #7029, #2282, .T. ) ;
#6761=DIRECTION ( 'NONE',  ( 1.000000000000000000, 0.000000000000000000, 9.776117811460147207E-16 ) ) ;
#6762=ADVANCED_FACE ( 'NONE', ( #6252, #2225, #6197 ), #4607, .F. ) ;
#6765=CARTESIAN_POINT ( 'NONE',  ( -2.293506896408097795, 120.5696653505793705, -16.00000000000000711 ) ) ;
#6767=ORIENTED_EDGE ( 'NONE', *, *, #7033, .T. ) ;
#6768=CARTESIAN_POINT ( 'NONE',  ( 53.40242741783141156, 52.77167129626698028, 25.00000000000000000 ) ) ;
#6769=ORIENTED_EDGE ( 'NONE', *, *, #2429, .T. ) ;
#6771=DIRECTION ( 'NONE',  ( 0.000000000000000000, -0.000000000000000000, 1.000000000000000000 ) ) ;
#6778=ORIENTED_EDGE ( 'NONE', *, *, #10013, .F. ) ;
#6779=EDGE_LOOP ( 'NONE', ( #5898, #9164, #6541, #8356 ) ) ;
#6782=CARTESIAN_POINT ( 'NONE',  ( -50.00000000000002132, -133.6308916829187581, 23.64290342185648797 ) ) ;
#6785=ORIENTED_EDGE ( 'NONE', *, *, #3566, .T. ) ;
#6786=CARTESIAN_POINT ( 'NONE',  ( -50.00000000000002132, -117.1457019118819005, -6.938893903907231533E-15 ) ) ;
#6787=ORIENTED_EDGE ( 'NONE', *, *, #2859, .T. ) ;
#6789=EDGE_CURVE ( 'NONE', #1658, #1605, #6971, .T. ) ;
#6792=ORIENTED_EDGE ( 'NONE', *, *, #1709, .T. ) ;
#6795=CARTESIAN_POINT ( 'NONE',  ( -25.15769640663940265, -133.1457019118818721, -3.513494341946491635E-15 ) ) ;
#6796=CARTESIAN_POINT ( 'NONE',  ( -25.15769640663938134, -115.1457019118818863, -48.00000000000002132 ) ) ;
#6800=ORIENTED_EDGE ( 'NONE', *, *, #6789, .T. ) ;
#6801=DIRECTION ( 'NONE',  ( 1.000000000000000000, 0.000000000000000000, -0.000000000000000000 ) ) ;
#6802=ORIENTED_EDGE ( 'NONE', *, *, #2859, .F. ) ;
#6805=DIRECTION ( 'NONE',  ( -0.000000000000000000, 1.000000000000000000, -0.000000000000000000 ) ) ;
#6806=AXIS2_PLACEMENT_3D ( 'NONE', #1893, #6022, #1260 ) ;
#6815=VECTOR ( 'NONE', #9844, 1000.000000000000000 ) ;
#6816=ORIENTED_EDGE ( 'NONE', *, *, #2489, .F. ) ;
#6818=CARTESIAN_POINT ( 'NONE',  ( 10.51964330236497602, 150.0000000000000000, -24.99999999999998934 ) ) ;
#6823=DIRECTION ( 'NONE',  ( 0.000000000000000000, 0.000000000000000000, 1.000000000000000000 ) ) ;
#6827=CARTESIAN_POINT ( 'NONE',  ( -40.00000000000002842, -135.1457019118818721, 39.99999999999997868 ) ) ;
#6830=CARTESIAN_POINT ( 'NONE',  ( -48.00000000000002132, -133.1457019118818721, 25.15769640663938134 ) ) ;
#6832=EDGE_LOOP ( 'NONE', ( #7107, #3295, #1216, #3792, #4995, #4711, #3104 ) ) ;
#6833=AXIS2_PLACEMENT_3D ( 'NONE', #1741, #4965, #9376 ) ;
#6835=EDGE_CURVE ( 'NONE', #1563, #5352, #6295, .T. ) ;
#6836=ADVANCED_FACE ( 'NONE', ( #7002 ), #7640, .T. ) ;
#6846=VERTEX_POINT ( 'NONE', #7462 ) ;
#6847=LINE ( 'NONE', #5249, #1348 ) ;
#6848=VECTOR ( 'NONE', #6225, 1000.000000000000000 ) ;
#6849=VERTEX_POINT ( 'NONE', #3435 ) ;
#6850=EDGE_CURVE ( 'NONE', #2017, #2630, #8043, .T. ) ;
#6853=DIRECTION ( 'NONE',  ( 0.000000000000000000, 0.000000000000000000, 1.000000000000000000 ) ) ;
#6854=CARTESIAN_POINT ( 'NONE',  ( -2.293506896408097795, 80.56966535057935630, 24.00000000000000711 ) ) ;
#6856=CARTESIAN_POINT ( 'NONE',  ( 37.22759939293836595, -133.1457019118818721, -25.15769640663939910 ) ) ;
#6857=AXIS2_PLACEMENT_3D ( 'NONE', #4030, #7263, #10446 ) ;
#6860=AXIS2_PLACEMENT_3D ( 'NONE', #8991, #9907, #7402 ) ;
#6862=CARTESIAN_POINT ( 'NONE',  ( 23.15769640663936713, -133.1457019118818721, 49.99999999999997868 ) ) ;
#6866=EDGE_CURVE ( 'NONE', #5250, #7894, #4600, .T. ) ;
#6867=CARTESIAN_POINT ( 'NONE',  ( 25.15769640663935292, -115.1457019118818863, 2.459446039362539254E-14 ) ) ;
#6869=VERTEX_POINT ( 'NONE', #4128 ) ;
#6870=CARTESIAN_POINT ( 'NONE',  ( 14.70649310359190309, 120.5696653505793705, -20.00000000000000711 ) ) ;
#6871=VECTOR ( 'NONE', #1869, 1000.000000000000000 ) ;
#6873=ORIENTED_EDGE ( 'NONE', *, *, #3096, .T. ) ;
#6876=ORIENTED_EDGE ( 'NONE', *, *, #8261, .T. ) ;
#6878=CYLINDRICAL_SURFACE ( 'NONE', #990, 10.00000000000000178 ) ;
#6879=PLANE ( 'NONE',  #2906 ) ;
#6881=LINE ( 'NONE', #4494, #1851 ) ;
#6882=DIRECTION ( 'NONE',  ( -0.000000000000000000, -0.000000000000000000, 1.000000000000000000 ) ) ;
#6884=VECTOR ( 'NONE', #1449, 1000.000000000000000 ) ;
#6885=CARTESIAN_POINT ( 'NONE',  ( 39.99999999999997158, -135.1457019118818721, 39.99999999999997868 ) ) ;
#6886=EDGE_CURVE ( 'NONE', #5017, #979, #37, .T. ) ;
#6889=AXIS2_PLACEMENT_3D ( 'NONE', #6768, #7512, #262 ) ;
#6890=DIRECTION ( 'NONE',  ( -0.000000000000000000, 1.000000000000000000, -0.000000000000000000 ) ) ;
#6893=CARTESIAN_POINT ( 'NONE',  ( -48.00000000000002132, -117.1457019118819005, -23.15769640663945594 ) ) ;
#6894=( LENGTH_UNIT ( ) NAMED_UNIT ( * ) SI_UNIT ( .MILLI., .METRE. ) );
#6895=CARTESIAN_POINT ( 'NONE',  ( 23.15769640663936713, -115.1457019118818863, 47.99999999999997868 ) ) ;
#6896=DIRECTION ( 'NONE',  ( 1.000000000000000000, 0.000000000000000000, -0.000000000000000000 ) ) ;
#6899=ADVANCED_FACE ( 'NONE', ( #8205 ), #102, .T. ) ;
#6900=EDGE_CURVE ( 'NONE', #4047, #9459, #943, .T. ) ;
#6901=ORIENTED_EDGE ( 'NONE', *, *, #2200, .T. ) ;
#6902=CONICAL_SURFACE ( 'NONE', #5703, 4.025000000000000355, 0.7853981633975870569 ) ;
#6906=ORIENTED_EDGE ( 'NONE', *, *, #4374, .T. ) ;
#6908=DIRECTION ( 'NONE',  ( 0.000000000000000000, 0.000000000000000000, 1.000000000000000000 ) ) ;
#6910=DIRECTION ( 'NONE',  ( 0.7525569905852205199, 0.6585271261848794078, 0.000000000000000000 ) ) ;
#6918=ORIENTED_EDGE ( 'NONE', *, *, #1293, .T. ) ;
#6919=CIRCLE ( 'NONE', #1288, 19.24539146688411506 ) ;
#6920=CARTESIAN_POINT ( 'NONE',  ( -25.15769640663937423, -133.1457019118818721, -48.00000000000002132 ) ) ;
#6921=AXIS2_PLACEMENT_3D ( 'NONE', #8608, #2139, #453 ) ;
#6922=DIRECTION ( 'NONE',  ( 9.776117811460147207E-16, 0.000000000000000000, -1.000000000000000000 ) ) ;
#6937=DIRECTION ( 'NONE',  ( 0.000000000000000000, 0.000000000000000000, 1.000000000000000000 ) ) ;
#6945=VERTEX_POINT ( 'NONE', #4807 ) ;
#6946=ADVANCED_FACE ( 'NONE', ( #161 ), #6612, .T. ) ;
#6947=CARTESIAN_POINT ( 'NONE',  ( 59.99999999999999289, -135.1457019118818721, -30.00000000000000355 ) ) ;
#6948=DIRECTION ( 'NONE',  ( 1.000000000000000000, 0.000000000000000000, 0.000000000000000000 ) ) ;
#6953=EDGE_LOOP ( 'NONE', ( #5764, #5134, #635, #1962 ) ) ;
#6955=ORIENTED_EDGE ( 'NONE', *, *, #7290, .F. ) ;
#6957=CARTESIAN_POINT ( 'NONE',  ( -40.00000000000002842, -135.1457019118818721, 35.99999999999999289 ) ) ;
#6958=DIRECTION ( 'NONE',  ( -1.000000000000000000, -0.000000000000000000, 0.000000000000000000 ) ) ;
#6961=DIRECTION ( 'NONE',  ( 0.000000000000000000, -1.000000000000000000, 0.000000000000000000 ) ) ;
#6962=DIRECTION ( 'NONE',  ( 1.000000000000000000, -0.000000000000000000, -0.000000000000000000 ) ) ;
#6963=FACE_OUTER_BOUND ( 'NONE', #8433, .T. ) ;
#6964=ORIENTED_EDGE ( 'NONE', *, *, #7290, .T. ) ;
#6965=DIRECTION ( 'NONE',  ( 0.000000000000000000, 0.000000000000000000, 1.000000000000000000 ) ) ;
#6966=FACE_OUTER_BOUND ( 'NONE', #8140, .T. ) ;
#6968=DIRECTION ( 'NONE',  ( 1.396588258780021135E-16, 0.000000000000000000, 1.000000000000000000 ) ) ;
#6969=ADVANCED_FACE ( 'NONE', ( #2478 ), #6879, .F. ) ;
#6970=ADVANCED_FACE ( 'NONE', ( #8416 ), #6078, .T. ) ;
#6971=CIRCLE ( 'NONE', #538, 4.000000000000000000 ) ;
#6974=DIRECTION ( 'NONE',  ( -1.734723475976805319E-15, 0.000000000000000000, 1.000000000000000000 ) ) ;
#6977=CARTESIAN_POINT ( 'NONE',  ( 37.59878849545336976, 32.08684478514406635, 30.00000000000000355 ) ) ;
#6978=ORIENTED_EDGE ( 'NONE', *, *, #5919, .T. ) ;
#6981=DIRECTION ( 'NONE',  ( -0.000000000000000000, 1.000000000000000000, -0.000000000000000000 ) ) ;
#6983=ORIENTED_EDGE ( 'NONE', *, *, #142, .F. ) ;
#6986=DIRECTION ( 'NONE',  ( 0.000000000000000000, 0.000000000000000000, -1.000000000000000000 ) ) ;
#6987=FACE_OUTER_BOUND ( 'NONE', #3831, .T. ) ;
#6988=ORIENTED_EDGE ( 'NONE', *, *, #6186, .F. ) ;
#6990=CARTESIAN_POINT ( 'NONE',  ( 39.99999999999997158, -135.1707019118818778, 39.99999999999997868 ) ) ;
#6991=DIRECTION ( 'NONE',  ( -0.07334937666141773394, 0.9973063064792990762, 0.000000000000000000 ) ) ;
#6992=VECTOR ( 'NONE', #8178, 1000.000000000000114 ) ;
#6993=CYLINDRICAL_SURFACE ( 'NONE', #2222, 10.00000000000000178 ) ;
#6994=CIRCLE ( 'NONE', #4920, 1.999999999999998224 ) ;
#6995=PLANE ( 'NONE',  #3681 ) ;
#6997=ORIENTED_EDGE ( 'NONE', *, *, #3937, .T. ) ;
#6998=CARTESIAN_POINT ( 'NONE',  ( -24.15108826162070699, -134.0910007290636941, -50.00000000000001421 ) ) ;
#6999=AXIS2_PLACEMENT_3D ( 'NONE', #3769, #7004, #2756 ) ;
#7002=FACE_OUTER_BOUND ( 'NONE', #3934, .T. ) ;
#7003=EDGE_LOOP ( 'NONE', ( #7390, #1900, #5662, #10245 ) ) ;
#7004=DIRECTION ( 'NONE',  ( -0.000000000000000000, -0.000000000000000000, 1.000000000000000000 ) ) ;
#7007=ORIENTED_EDGE ( 'NONE', *, *, #746, .F. ) ;
#7011=AXIS2_PLACEMENT_3D ( 'NONE', #9554, #4719, #1381 ) ;
#7013=ORIENTED_EDGE ( 'NONE', *, *, #8185, .F. ) ;
#7015=CARTESIAN_POINT ( 'NONE',  ( 37.22511195853869026, -115.1457019118818863, 0.000000000000000000 ) ) ;
#7020=ORIENTED_EDGE ( 'NONE', *, *, #5367, .F. ) ;
#7021=CARTESIAN_POINT ( 'NONE',  ( 14.70649310359190309, 80.56966535057935630, 24.00000000000000711 ) ) ;
#7023=CIRCLE ( 'NONE', #2777, 5.000000000000000888 ) ;
#7024=ORIENTED_EDGE ( 'NONE', *, *, #8613, .F. ) ;
#7027=CARTESIAN_POINT ( 'NONE',  ( -27.15769640663940976, -115.1457019118818863, 25.15769640663938134 ) ) ;
#7029=VERTEX_POINT ( 'NONE', #10062 ) ;
#7033=EDGE_CURVE ( 'NONE', #6120, #4912, #9004, .T. ) ;
#7038=VERTEX_POINT ( 'NONE', #5232 ) ;
#7039=ORIENTED_EDGE ( 'NONE', *, *, #6603, .F. ) ;
#7042=ORIENTED_EDGE ( 'NONE', *, *, #7426, .T. ) ;
#7045=CARTESIAN_POINT ( 'NONE',  ( 80.08610854271790913, 54.73418909528891874, 30.00000000000000355 ) ) ;
#7046=CARTESIAN_POINT ( 'NONE',  ( -48.00000000000002132, -117.1457019118819005, 23.15769640663938134 ) ) ;
#7051=VERTEX_POINT ( 'NONE', #3649 ) ;
#7055=CARTESIAN_POINT ( 'NONE',  ( 39.99999999999998579, -135.1707019118818778, -40.00000000000002132 ) ) ;
#7056=DIRECTION ( 'NONE',  ( 0.000000000000000000, -1.000000000000000000, 0.000000000000000000 ) ) ;
#7057=AXIS2_PLACEMENT_3D ( 'NONE', #4472, #7602, #5050 ) ;
#7058=CARTESIAN_POINT ( 'NONE',  ( -2.293506896408097795, 152.5696653505793279, 30.00000000000000355 ) ) ;
#7059=FACE_OUTER_BOUND ( 'NONE', #4626, .T. ) ;
#7063=EDGE_LOOP ( 'NONE', ( #3152, #4915, #649, #4839 ) ) ;
#7068=EDGE_CURVE ( 'NONE', #8567, #7162, #881, .T. ) ;
#7069=DIRECTION ( 'NONE',  ( 0.000000000000000000, -1.000000000000000000, 0.000000000000000000 ) ) ;
#7071=LINE ( 'NONE', #3036, #4168 ) ;
#7074=DIRECTION ( 'NONE',  ( 1.000000000000000000, 0.000000000000000000, 0.000000000000000000 ) ) ;
#7075=ORIENTED_EDGE ( 'NONE', *, *, #8077, .F. ) ;
#7078=VERTEX_POINT ( 'NONE', #7673 ) ;
#7082=VECTOR ( 'NONE', #3676, 1000.000000000000000 ) ;
#7085=DIRECTION ( 'NONE',  ( 1.000000000000000000, 0.000000000000000000, 0.000000000000000000 ) ) ;
#7088=DIRECTION ( 'NONE',  ( 0.000000000000000000, 1.000000000000000000, 0.000000000000000000 ) ) ;
#7090=AXIS2_PLACEMENT_3D ( 'NONE', #9385, #10181, #5294 ) ;
#7093=EDGE_LOOP ( 'NONE', ( #6286, #8253, #6964, #2584 ) ) ;
#7097=EDGE_CURVE ( 'NONE', #9778, #732, #8835, .T. ) ;
#7098=EDGE_CURVE ( 'NONE', #9534, #86, #8669, .T. ) ;
#7099=FACE_OUTER_BOUND ( 'NONE', #2393, .T. ) ;
#7100=DIRECTION ( 'NONE',  ( 0.000000000000000000, 0.000000000000000000, 1.000000000000000000 ) ) ;
#7102=DIRECTION ( 'NONE',  ( 0.000000000000000000, -0.000000000000000000, 1.000000000000000000 ) ) ;
#7104=AXIS2_PLACEMENT_3D ( 'NONE', #1928, #10045, #8399 ) ;
#7105=VERTEX_POINT ( 'NONE', #9213 ) ;
#7107=ORIENTED_EDGE ( 'NONE', *, *, #10280, .F. ) ;
#7111=EDGE_CURVE ( 'NONE', #2586, #6030, #2268, .T. ) ;
#7113=VERTEX_POINT ( 'NONE', #10331 ) ;
#7116=DIRECTION ( 'NONE',  ( 0.000000000000000000, 0.000000000000000000, 1.000000000000000000 ) ) ;
#7117=DIRECTION ( 'NONE',  ( -1.000000000000000000, 0.000000000000000000, -0.000000000000000000 ) ) ;
#7118=EDGE_LOOP ( 'NONE', ( #1257, #4005, #6876, #69 ) ) ;
#7119=ORIENTED_EDGE ( 'NONE', *, *, #8315, .F. ) ;
#7121=EDGE_LOOP ( 'NONE', ( #1411, #5476, #1139 ) ) ;
#7122=LINE ( 'NONE', #2187, #2337 ) ;
#7123=CARTESIAN_POINT ( 'NONE',  ( 37.22511195853866894, 17.84145331825995839, -24.99999999999998934 ) ) ;
#7124=PLANE ( 'NONE',  #8571 ) ;
#7126=DIRECTION ( 'NONE',  ( 0.000000000000000000, -0.000000000000000000, -1.000000000000000000 ) ) ;
#7130=VERTEX_POINT ( 'NONE', #4052 ) ;
#7131=DIRECTION ( 'NONE',  ( 0.000000000000000000, 0.000000000000000000, -1.000000000000000000 ) ) ;
#7135=CARTESIAN_POINT ( 'NONE',  ( -48.00000000000002132, -117.1457019118819005, -23.15769640663945594 ) ) ;
#7136=EDGE_LOOP ( 'NONE', ( #8784, #4904, #927, #6675 ) ) ;
#7140=VERTEX_POINT ( 'NONE', #1420 ) ;
#7145=EDGE_LOOP ( 'NONE', ( #5704, #8593, #4483, #5615 ) ) ;
#7149=FACE_OUTER_BOUND ( 'NONE', #4660, .T. ) ;
#7151=DIRECTION ( 'NONE',  ( 0.000000000000000000, 0.000000000000000000, 1.000000000000000000 ) ) ;
#7152=AXIS2_PLACEMENT_3D ( 'NONE', #4834, #815, #2104 ) ;
#7153=EDGE_CURVE ( 'NONE', #3513, #7537, #7316, .T. ) ;
#7155=CARTESIAN_POINT ( 'NONE',  ( -25.15769640663939199, -133.1457019118818721, -27.15769640663944173 ) ) ;
#7157=DIRECTION ( 'NONE',  ( 0.000000000000000000, 0.000000000000000000, 1.000000000000000000 ) ) ;
#7162=VERTEX_POINT ( 'NONE', #3863 ) ;
#7165=EDGE_CURVE ( 'NONE', #9778, #6079, #5680, .T. ) ;
#7166=CIRCLE ( 'NONE', #8004, 2.525240063345735475 ) ;
#7169=CARTESIAN_POINT ( 'NONE',  ( -16.29350689640809691, -186.9457019118818835, 7.500000000000000000 ) ) ;
#7170=DIRECTION ( 'NONE',  ( -1.000000000000000000, -0.000000000000000000, 0.000000000000000000 ) ) ;
#7175=DIRECTION ( 'NONE',  ( 0.000000000000000000, -1.000000000000000000, 0.000000000000000000 ) ) ;
#7181=CARTESIAN_POINT ( 'NONE',  ( -16.29350689640809691, -115.1457019118818863, -30.31717237747080773 ) ) ;
#7183=FACE_OUTER_BOUND ( 'NONE', #2991, .T. ) ;
#7186=ORIENTED_EDGE ( 'NONE', *, *, #6644, .F. ) ;
#7187=FACE_OUTER_BOUND ( 'NONE', #10350, .T. ) ;
#7190=CARTESIAN_POINT ( 'NONE',  ( -2.293506896408094242, 37.08684478514405214, -12.50000000000000000 ) ) ;
#7191=VERTEX_POINT ( 'NONE', #9728 ) ;
#7192=AXIS2_PLACEMENT_3D ( 'NONE', #5682, #8235, #8125 ) ;
#7194=LINE ( 'NONE', #9478, #1623 ) ;
#7195=EDGE_CURVE ( 'NONE', #8587, #2261, #3751, .T. ) ;
#7196=DIRECTION ( 'NONE',  ( -1.000000000000000000, 0.000000000000000000, 0.000000000000000000 ) ) ;
#7200=FACE_OUTER_BOUND ( 'NONE', #7121, .T. ) ;
#7203=DIRECTION ( 'NONE',  ( -6.982941293900105430E-16, 0.000000000000000000, 1.000000000000000000 ) ) ;
#7205=CYLINDRICAL_SURFACE ( 'NONE', #8943, 2.000000000000001776 ) ;
#7206=DIRECTION ( 'NONE',  ( 0.000000000000000000, 0.000000000000000000, 1.000000000000000000 ) ) ;
#7208=EDGE_CURVE ( 'NONE', #4536, #6699, #8675, .T. ) ;
#7210=AXIS2_PLACEMENT_3D ( 'NONE', #2311, #8718, #2939 ) ;
#7211=FACE_OUTER_BOUND ( 'NONE', #6430, .T. ) ;
#7212=ORIENTED_EDGE ( 'NONE', *, *, #6835, .T. ) ;
#7215=CIRCLE ( 'NONE', #7387, 7.525240063345735031 ) ;
#7219=CARTESIAN_POINT ( 'NONE',  ( -20.14472382240651882, -141.8229441850657793, -25.87097612368021160 ) ) ;
#7221=ADVANCED_FACE ( 'NONE', ( #6987 ), #7885, .F. ) ;
#7223=EDGE_CURVE ( 'NONE', #1967, #9556, #79, .T. ) ;
#7224=CARTESIAN_POINT ( 'NONE',  ( -27.15769640663937778, -135.1457019118818721, -48.00000000000002132 ) ) ;
#7232=ADVANCED_FACE ( 'NONE', ( #6182 ), #1366, .T. ) ;
#7246=CARTESIAN_POINT ( 'NONE',  ( 14.70649310359190309, 80.56966535057935630, -24.00000000000000711 ) ) ;
#7247=CARTESIAN_POINT ( 'NONE',  ( 4.856471286862175774, 152.5696653505793279, -25.00000000000001776 ) ) ;
#7249=DIRECTION ( 'NONE',  ( 1.000000000000000000, 0.000000000000000000, 0.000000000000000000 ) ) ;
#7252=ADVANCED_FACE ( 'NONE', ( #2714 ), #1075, .T. ) ;
#7253=ORIENTED_EDGE ( 'NONE', *, *, #3167, .F. ) ;
#7254=CARTESIAN_POINT ( 'NONE',  ( -27.15769640663939555, -135.1457019118818721, -25.15769640663944173 ) ) ;
#7256=EDGE_CURVE ( 'NONE', #7422, #7140, #5153, .T. ) ;
#7259=VECTOR ( 'NONE', #6611, 1000.000000000000000 ) ;
#7260=CARTESIAN_POINT ( 'NONE',  ( -23.76520584195948516, -145.1457019118819005, -97.78965767959371647 ) ) ;
#7262=DIRECTION ( 'NONE',  ( -0.000000000000000000, 1.000000000000000000, -0.000000000000000000 ) ) ;
#7263=DIRECTION ( 'NONE',  ( -0.000000000000000000, -1.000000000000000000, -0.000000000000000000 ) ) ;
#7266=ORIENTED_EDGE ( 'NONE', *, *, #2091, .F. ) ;
#7267=EDGE_CURVE ( 'NONE', #640, #2261, #9178, .T. ) ;
#7268=EDGE_LOOP ( 'NONE', ( #2232, #4091, #5149 ) ) ;
#7271=DIRECTION ( 'NONE',  ( 0.000000000000000000, 0.000000000000000000, -1.000000000000000000 ) ) ;
#7273=VERTEX_POINT ( 'NONE', #9029 ) ;
#7274=LINE ( 'NONE', #5775, #1479 ) ;
#7279=VERTEX_POINT ( 'NONE', #7601 ) ;
#7280=FACE_OUTER_BOUND ( 'NONE', #7093, .T. ) ;
#7283=CARTESIAN_POINT ( 'NONE',  ( -40.00000000000001421, -135.1457019118818721, -35.97500000000002274 ) ) ;
#7284=ORIENTED_EDGE ( 'NONE', *, *, #10280, .T. ) ;
#7285=CARTESIAN_POINT ( 'NONE',  ( -16.29350689640809691, -186.9457019118818835, 27.01918567566963247 ) ) ;
#7287=ADVANCED_FACE ( 'NONE', ( #5942 ), #8977, .T. ) ;
#7289=EDGE_CURVE ( 'NONE', #6699, #2391, #4766, .T. ) ;
#7290=EDGE_CURVE ( 'NONE', #996, #4419, #2667, .T. ) ;
#7292=ORIENTED_EDGE ( 'NONE', *, *, #618, .F. ) ;
#7293=LINE ( 'NONE', #6604, #8583 ) ;
#7294=AXIS2_PLACEMENT_3D ( 'NONE', #6292, #2369, #7249 ) ;
#7295=CARTESIAN_POINT ( 'NONE',  ( -23.76520584195948516, -145.1457019118819005, -0.6509338422960262438 ) ) ;
#7297=CARTESIAN_POINT ( 'NONE',  ( -23.15769640663940976, -115.1457019118818863, 47.99999999999997868 ) ) ;
#7304=VERTEX_POINT ( 'NONE', #5790 ) ;
#7309=EDGE_CURVE ( 'NONE', #2474, #9955, #2400, .T. ) ;
#7310=CARTESIAN_POINT ( 'NONE',  ( 23.15769640663936713, -115.1457019118818863, 49.99999999999997868 ) ) ;
#7311=AXIS2_PLACEMENT_3D ( 'NONE', #3222, #4961, #5814 ) ;
#7316=CIRCLE ( 'NONE', #3935, 1.999999999999998224 ) ;
#7317=ORIENTED_EDGE ( 'NONE', *, *, #8765, .F. ) ;
#7318=VECTOR ( 'NONE', #2093, 1000.000000000000000 ) ;
#7325=B_SPLINE_CURVE_WITH_KNOTS ( 'NONE', 3,
 ( #10238, #1171, #2970, #6200, #9443, #5138, #3559, #6782, #4349, #4404 ),
 .UNSPECIFIED., .F., .F.,
 ( 4, 2, 2, 2, 4 ),
 ( 0.000000000000000000, 0.001023740819106953685, 0.002047481638213907371, 0.003071222457320861056, 0.004094963276427814741 ),
 .UNSPECIFIED. ) ;
#7326=DIRECTION ( 'NONE',  ( 0.9973063064792990762, 0.07334937666141773394, 0.000000000000000000 ) ) ;
#7327=EDGE_CURVE ( 'NONE', #3326, #7029, #5114, .T. ) ;
#7333=CARTESIAN_POINT ( 'NONE',  ( -50.00000000000002132, -133.1457019118818721, -23.15769640663945594 ) ) ;
#7335=DIRECTION ( 'NONE',  ( -0.000000000000000000, 0.000000000000000000, 1.000000000000000000 ) ) ;
#7336=EDGE_CURVE ( 'NONE', #9783, #6462, #3465, .T. ) ;
#7337=DIRECTION ( 'NONE',  ( 0.000000000000000000, 0.000000000000000000, 1.000000000000000000 ) ) ;
#7338=ORIENTED_EDGE ( 'NONE', *, *, #6900, .T. ) ;
#7339=CARTESIAN_POINT ( 'NONE',  ( -23.15769640663939199, -117.1457019118819005, -27.15769640663944173 ) ) ;
#7340=CIRCLE ( 'NONE', #1919, 2.525240063345735475 ) ;
#7342=CARTESIAN_POINT ( 'NONE',  ( -24.98777100551300023, -134.6884840344297913, 49.99999999999998579 ) ) ;
#7343=ORIENTED_EDGE ( 'NONE', *, *, #3149, .T. ) ;
#7344=VERTEX_POINT ( 'NONE', #4257 ) ;
#7346=CARTESIAN_POINT ( 'NONE',  ( -23.48622939173158386, -144.8896666241527669, -3.853145670227909658 ) ) ;
#7347=EDGE_CURVE ( 'NONE', #9534, #1811, #4208, .T. ) ;
#7351=EDGE_CURVE ( 'NONE', #7113, #8587, #6643, .T. ) ;
#7352=SPHERICAL_SURFACE ( 'NONE', #5259, 2.000000000000000000 ) ;
#7355=CIRCLE ( 'NONE', #7192, 24.24539146688411861 ) ;
#7357=VERTEX_POINT ( 'NONE', #9994 ) ;
#7358=DIRECTION ( 'NONE',  ( 1.000000000000000000, 0.000000000000000000, 0.000000000000000000 ) ) ;
#7360=CARTESIAN_POINT ( 'NONE',  ( 42.22511195853868315, -135.1457019118818721, 25.00000000000000000 ) ) ;
#7363=VECTOR ( 'NONE', #842, 1000.000000000000114 ) ;
#7366=ORIENTED_EDGE ( 'NONE', *, *, #995, .T. ) ;
#7367=ORIENTED_EDGE ( 'NONE', *, *, #7542, .T. ) ;
#7368=ORIENTED_EDGE ( 'NONE', *, *, #3849, .T. ) ;
#7369=EDGE_LOOP ( 'NONE', ( #6571, #6633, #5515, #6800 ) ) ;
#7371=AXIS2_PLACEMENT_3D ( 'NONE', #2272, #4705, #5552 ) ;
#7373=CARTESIAN_POINT ( 'NONE',  ( 37.59878849545336976, 37.08684478514406635, 12.50000000000000711 ) ) ;
#7380=ORIENTED_EDGE ( 'NONE', *, *, #6310, .T. ) ;
#7382=CARTESIAN_POINT ( 'NONE',  ( -2.293506896408097795, 37.08684478514406635, 30.00000000000000355 ) ) ;
#7383=DIRECTION ( 'NONE',  ( 0.000000000000000000, -1.000000000000000000, 0.000000000000000000 ) ) ;
#7387=AXIS2_PLACEMENT_3D ( 'NONE', #4785, #9841, #3306 ) ;
#7390=ORIENTED_EDGE ( 'NONE', *, *, #3538, .F. ) ;
#7391=FACE_OUTER_BOUND ( 'NONE', #8654, .T. ) ;
#7392=AXIS2_PLACEMENT_3D ( 'NONE', #7722, #1362, #1254 ) ;
#7395=CARTESIAN_POINT ( 'NONE',  ( -24.15110854952566299, -134.0910177696405299, 49.99999999999997868 ) ) ;
#7396=EDGE_CURVE ( 'NONE', #9491, #3983, #720, .T. ) ;
#7397=ORIENTED_EDGE ( 'NONE', *, *, #817, .T. ) ;
#7399=VECTOR ( 'NONE', #7539, 1000.000000000000000 ) ;
#7402=DIRECTION ( 'NONE',  ( 0.000000000000000000, -0.000000000000000000, -1.000000000000000000 ) ) ;
#7408=CARTESIAN_POINT ( 'NONE',  ( -18.34874108452141783, -140.1746510883711778, -97.78965767959371647 ) ) ;
#7417=DIRECTION ( 'NONE',  ( -1.000000000000000000, 0.000000000000000000, -8.379529552680124346E-16 ) ) ;
#7418=AXIS2_PLACEMENT_3D ( 'NONE', #3121, #3820, #9656 ) ;
#7420=DIRECTION ( 'NONE',  ( 0.000000000000000000, 0.000000000000000000, 1.000000000000000000 ) ) ;
#7421=VERTEX_POINT ( 'NONE', #6854 ) ;
#7422=VERTEX_POINT ( 'NONE', #9399 ) ;
#7423=EDGE_CURVE ( 'NONE', #6261, #6849, #7997, .T. ) ;
#7426=EDGE_CURVE ( 'NONE', #7523, #4871, #1905, .T. ) ;
#7427=DIRECTION ( 'NONE',  ( -0.000000000000000000, 1.000000000000000000, 0.000000000000000000 ) ) ;
#7431=ORIENTED_EDGE ( 'NONE', *, *, #6125, .F. ) ;
#7439=FACE_BOUND ( 'NONE', #6620, .T. ) ;
#7441=DIRECTION ( 'NONE',  ( -0.000000000000000000, -0.000000000000000000, -1.000000000000000000 ) ) ;
#7443=DIRECTION ( 'NONE',  ( -1.000000000000000000, -0.000000000000000000, -8.379529552680125332E-16 ) ) ;
#7445=DIRECTION ( 'NONE',  ( 0.000000000000000000, 0.000000000000000000, 1.000000000000000000 ) ) ;
#7450=CARTESIAN_POINT ( 'NONE',  ( -48.00000000000002132, -117.1457019118819005, 25.15769640663938134 ) ) ;
#7451=EDGE_LOOP ( 'NONE', ( #9560, #4630, #9227, #10180 ) ) ;
#7454=DIRECTION ( 'NONE',  ( 0.000000000000000000, 0.000000000000000000, -1.000000000000000000 ) ) ;
#7456=DIRECTION ( 'NONE',  ( -1.000000000000000000, -0.000000000000000000, -0.000000000000000000 ) ) ;
#7457=CARTESIAN_POINT ( 'NONE',  ( -40.00000000000002842, -135.1457019118818721, 39.99999999999997868 ) ) ;
#7459=ORIENTED_EDGE ( 'NONE', *, *, #1275, .T. ) ;
#7461=ORIENTED_EDGE ( 'NONE', *, *, #10385, .F. ) ;
#7462=CARTESIAN_POINT ( 'NONE',  ( 25.15769640663940265, -117.1457019118819005, -48.00000000000002132 ) ) ;
#7463=LINE ( 'NONE', #999, #9821 ) ;
#7464=DIRECTION ( 'NONE',  ( 1.000000000000000000, 0.000000000000000000, 0.000000000000000000 ) ) ;
#7465=CARTESIAN_POINT ( 'NONE',  ( -18.34874108452141783, -140.1746510883711778, 49.99999999999997868 ) ) ;
#7466=DIRECTION ( 'NONE',  ( 0.000000000000000000, 1.000000000000000000, 0.000000000000000000 ) ) ;
#7467=EDGE_CURVE ( 'NONE', #172, #1886, #2132, .T. ) ;
#7477=DIRECTION ( 'NONE',  ( 1.000000000000000000, 0.000000000000000000, 0.000000000000000000 ) ) ;
#7480=EDGE_CURVE ( 'NONE', #4076, #4567, #557, .T. ) ;
#7482=ADVANCED_FACE ( 'NONE', ( #4572 ), #7803, .F. ) ;
#7484=VERTEX_POINT ( 'NONE', #1394 ) ;
#7489=PRODUCT_DEFINITION_CONTEXT ( 'detailed design', #770, 'design' ) ;
#7490=CARTESIAN_POINT ( 'NONE',  ( 23.15769640663936713, -133.1457019118818721, 47.99999999999997868 ) ) ;
#7491=CARTESIAN_POINT ( 'NONE',  ( 0.000000000000000000, -115.1457019118818863, 0.000000000000000000 ) ) ;
#7492=CARTESIAN_POINT ( 'NONE',  ( -40.00000000000002842, -135.1457019118818721, 39.99999999999997868 ) ) ;
#7493=DIRECTION ( 'NONE',  ( 1.000000000000000000, -0.000000000000000000, -0.000000000000000000 ) ) ;
#7496=CARTESIAN_POINT ( 'NONE',  ( -21.44003972449640116, -143.0117419471019673, 6.332076144530967454 ) ) ;
#7497=EDGE_CURVE ( 'NONE', #4536, #249, #5799, .T. ) ;
#7498=ORIENTED_EDGE ( 'NONE', *, *, #9553, .F. ) ;
#7502=DIRECTION ( 'NONE',  ( 1.000000000000000000, 0.000000000000000000, 0.000000000000000000 ) ) ;
#7508=CARTESIAN_POINT ( 'NONE',  ( 27.15769640663938489, -117.1457019118819005, -27.15769640663940976 ) ) ;
#7511=ORIENTED_EDGE ( 'NONE', *, *, #1915, .T. ) ;
#7512=DIRECTION ( 'NONE',  ( 0.000000000000000000, 0.000000000000000000, 1.000000000000000000 ) ) ;
#7515=CARTESIAN_POINT ( 'NONE',  ( -16.29350689640809691, -140.1746510883711778, 7.500000000000000000 ) ) ;
#7517=FACE_OUTER_BOUND ( 'NONE', #10400, .T. ) ;
#7522=VECTOR ( 'NONE', #1923, 1000.000000000000000 ) ;
#7523=VERTEX_POINT ( 'NONE', #7701 ) ;
#7524=EDGE_LOOP ( 'NONE', ( #671, #1086, #1486, #7823, #4714, #7292, #6545, #6787 ) ) ;
#7530=DIRECTION ( 'NONE',  ( -0.000000000000000000, 1.000000000000000000, -0.000000000000000000 ) ) ;
#7532=ORIENTED_EDGE ( 'NONE', *, *, #9293, .F. ) ;
#7534=ORIENTED_EDGE ( 'NONE', *, *, #5008, .T. ) ;
#7535=DIRECTION ( 'NONE',  ( 0.000000000000000000, 0.000000000000000000, 1.000000000000000000 ) ) ;
#7536=CIRCLE ( 'NONE', #7371, 3.999999999999996447 ) ;
#7537=VERTEX_POINT ( 'NONE', #752 ) ;
#7539=DIRECTION ( 'NONE',  ( -0.6585271261848804070, 0.7525569905852197428, 0.000000000000000000 ) ) ;
#7541=DIRECTION ( 'NONE',  ( 0.000000000000000000, 0.000000000000000000, -1.000000000000000000 ) ) ;
#7542=EDGE_CURVE ( 'NONE', #4047, #3180, #1651, .T. ) ;
#7543=DIRECTION ( 'NONE',  ( 0.000000000000000000, 0.000000000000000000, -1.000000000000000000 ) ) ;
#7547=VECTOR ( 'NONE', #8982, 1000.000000000000000 ) ;
#7548=ORIENTED_EDGE ( 'NONE', *, *, #5977, .F. ) ;
#7549=DIRECTION ( 'NONE',  ( -1.000000000000000000, 0.000000000000000000, -0.000000000000000000 ) ) ;
#7550=EDGE_LOOP ( 'NONE', ( #6016, #7338, #3210, #9417 ) ) ;
#7551=CIRCLE ( 'NONE', #4833, 5.000000000000000888 ) ;
#7556=ORIENTED_EDGE ( 'NONE', *, *, #9788, .T. ) ;
#7560=AXIS2_PLACEMENT_3D ( 'NONE', #2820, #10309, #9510 ) ;
#7563=CARTESIAN_POINT ( 'NONE',  ( -23.15769640663940976, -117.1457019118819005, 47.99999999999997868 ) ) ;
#7569=EDGE_LOOP ( 'NONE', ( #340, #5978, #9234, #9832 ) ) ;
#7571=DIRECTION ( 'NONE',  ( -1.000000000000000000, 0.000000000000000000, -0.000000000000000000 ) ) ;
#7572=CARTESIAN_POINT ( 'NONE',  ( 99.80027788547049283, -145.1457019118819005, 30.00000000000000355 ) ) ;
#7580=ORIENTED_EDGE ( 'NONE', *, *, #6644, .T. ) ;
#7581=VECTOR ( 'NONE', #906, 1000.000000000000000 ) ;
#7582=ORIENTED_EDGE ( 'NONE', *, *, #8703, .T. ) ;
#7583=DIRECTION ( 'NONE',  ( -1.000000000000000000, -0.000000000000000000, -0.000000000000000000 ) ) ;
#7584=CARTESIAN_POINT ( 'NONE',  ( 37.22511195853868315, -116.3672949040186779, -25.00000000000000355 ) ) ;
#7590=CARTESIAN_POINT ( 'NONE',  ( -27.15769640663940976, -115.1457019118818863, 23.15769640663938134 ) ) ;
#7594=CIRCLE ( 'NONE', #983, 2.000000000000001776 ) ;
#7595=ORIENTED_EDGE ( 'NONE', *, *, #5069, .T. ) ;
#7597=EDGE_LOOP ( 'NONE', ( #2049, #4582, #9470, #951 ) ) ;
#7599=CARTESIAN_POINT ( 'NONE',  ( 27.15769640663936713, -133.1457019118818721, 27.15769640663938489 ) ) ;
#7600=DIRECTION ( 'NONE',  ( -0.000000000000000000, 1.000000000000000000, 0.000000000000000000 ) ) ;
#7601=CARTESIAN_POINT ( 'NONE',  ( -48.00000000000002842, -115.1457019118818863, 23.15769640663938134 ) ) ;
#7602=DIRECTION ( 'NONE',  ( 0.000000000000000000, -1.000000000000000000, 0.000000000000000000 ) ) ;
#7603=ORIENTED_EDGE ( 'NONE', *, *, #6447, .T. ) ;
#7608=EDGE_LOOP ( 'NONE', ( #4592, #6631, #4868, #7842 ) ) ;
#7609=CARTESIAN_POINT ( 'NONE',  ( 2.108096605167896559E-14, -115.1457019118818863, -25.15769640663943107 ) ) ;
#7612=DIRECTION ( 'NONE',  ( 0.000000000000000000, 0.000000000000000000, 1.000000000000000000 ) ) ;
#7614=ORIENTED_EDGE ( 'NONE', *, *, #6759, .F. ) ;
#7615=CARTESIAN_POINT ( 'NONE',  ( -27.15769640663939555, -117.1457019118819005, -27.15769640663944173 ) ) ;
#7621=ORIENTED_EDGE ( 'NONE', *, *, #7098, .F. ) ;
#7624=DIRECTION ( 'NONE',  ( -8.379529552680124346E-16, 0.000000000000000000, 1.000000000000000000 ) ) ;
#7630=ORIENTED_EDGE ( 'NONE', *, *, #9849, .F. ) ;
#7632=DIRECTION ( 'NONE',  ( 1.000000000000000000, 0.000000000000000000, 0.000000000000000000 ) ) ;
#7634=CARTESIAN_POINT ( 'NONE',  ( -48.00000000000002132, -135.1457019118818721, -27.15769640663945950 ) ) ;
#7639=VERTEX_POINT ( 'NONE', #6370 ) ;
#7640=TOROIDAL_SURFACE ( 'NONE', #7649, 4.000000000000000000, 2.000000000000000000 ) ;
#7647=DIRECTION ( 'NONE',  ( -1.000000000000000000, 0.000000000000000000, -8.379529552680125332E-16 ) ) ;
#7648=PLANE ( 'NONE',  #449 ) ;
#7649=AXIS2_PLACEMENT_3D ( 'NONE', #2175, #7056, #10292 ) ;
#7650=ORIENTED_EDGE ( 'NONE', *, *, #118, .F. ) ;
#7652=LINE ( 'NONE', #2771, #10021 ) ;
#7653=ORIENTED_EDGE ( 'NONE', *, *, #7749, .F. ) ;
#7656=AXIS2_PLACEMENT_3D ( 'NONE', #3364, #2510, #972 ) ;
#7659=CARTESIAN_POINT ( 'NONE',  ( 39.99999999999998579, -135.1707019118818778, -44.00000000000002132 ) ) ;
#7668=ORIENTED_EDGE ( 'NONE', *, *, #8865, .T. ) ;
#7673=CARTESIAN_POINT ( 'NONE',  ( 42.22511195853868315, -135.1457019118818721, 30.00000000000000355 ) ) ;
#7676=LINE ( 'NONE', #1046, #9134 ) ;
#7679=CARTESIAN_POINT ( 'NONE',  ( 39.99999999999998579, -135.1457019118818721, -40.00000000000002132 ) ) ;
#7682=ORIENTED_EDGE ( 'NONE', *, *, #1026, .T. ) ;
#7687=CYLINDRICAL_SURFACE ( 'NONE', #3023, 4.000000000000000000 ) ;
#7689=EDGE_CURVE ( 'NONE', #9794, #415, #6136, .T. ) ;
#7691=DIRECTION ( 'NONE',  ( -0.6585271261848804070, 0.7525569905852197428, 0.000000000000000000 ) ) ;
#7692=CIRCLE ( 'NONE', #9564, 4.025000000000000355 ) ;
#7698=LINE ( 'NONE', #6049, #9796 ) ;
#7699=CARTESIAN_POINT ( 'NONE',  ( -23.15769640663940976, -115.1457019118818863, 49.99999999999997868 ) ) ;
#7701=CARTESIAN_POINT ( 'NONE',  ( 23.15769640663936357, -115.1457019118818863, 27.15769640663938489 ) ) ;
#7707=PLANE ( 'NONE',  #5568 ) ;
#7709=VECTOR ( 'NONE', #309, 1000.000000000000000 ) ;
#7711=CARTESIAN_POINT ( 'NONE',  ( 37.46742560152671331, -135.0531259799080033, 26.54270448881459643 ) ) ;
#7712=DIRECTION ( 'NONE',  ( -1.000000000000000000, -0.000000000000000000, -0.000000000000000000 ) ) ;
#7713=FACE_OUTER_BOUND ( 'NONE', #7819, .T. ) ;
#7717=ORIENTED_EDGE ( 'NONE', *, *, #757, .T. ) ;
#7721=VECTOR ( 'NONE', #6323, 1000.000000000000000 ) ;
#7722=CARTESIAN_POINT ( 'NONE',  ( -2.293506896408097795, 37.08684478514406635, 30.00000000000000355 ) ) ;
#7723=ORIENTED_EDGE ( 'NONE', *, *, #8806, .T. ) ;
#7725=DIRECTION ( 'NONE',  ( 0.000000000000000000, 1.000000000000000000, 0.000000000000000000 ) ) ;
#7727=VECTOR ( 'NONE', #8684, 1000.000000000000000 ) ;
#7729=LINE ( 'NONE', #323, #2424 ) ;
#7730=CARTESIAN_POINT ( 'NONE',  ( -27.15769640663940976, -133.1457019118818721, 27.15769640663938489 ) ) ;
#7731=VECTOR ( 'NONE', #2166, 1000.000000000000000 ) ;
#7739=MECHANICAL_DESIGN_GEOMETRIC_PRESENTATION_REPRESENTATION('',(#3509),#7909);
#7746=ORIENTED_EDGE ( 'NONE', *, *, #4655, .T. ) ;
#7748=EDGE_CURVE ( 'NONE', #7894, #3749, #1012, .T. ) ;
#7749=EDGE_CURVE ( 'NONE', #2514, #5655, #7166, .T. ) ;
#7752=ORIENTED_EDGE ( 'NONE', *, *, #5916, .F. ) ;
#7753=ORIENTED_EDGE ( 'NONE', *, *, #2429, .F. ) ;
#7755=CARTESIAN_POINT ( 'NONE',  ( -16.29350689640809691, -115.1457019118818863, 23.72119897386845722 ) ) ;
#7760=ORIENTED_EDGE ( 'NONE', *, *, #8952, .T. ) ;
#7761=CARTESIAN_POINT ( 'NONE',  ( -2.293506896408097795, 80.56966535057935630, 20.00000000000000711 ) ) ;
#7762=ADVANCED_FACE ( 'NONE', ( #2601 ), #228, .T. ) ;
#7763=DIRECTION ( 'NONE',  ( -9.776117811460147207E-16, 0.000000000000000000, 1.000000000000000000 ) ) ;
#7768=DIRECTION ( 'NONE',  ( -0.000000000000000000, 1.000000000000000000, -0.000000000000000000 ) ) ;
#7770=ORIENTED_EDGE ( 'NONE', *, *, #9304, .T. ) ;
#7771=DIRECTION ( 'NONE',  ( 0.000000000000000000, 0.000000000000000000, 1.000000000000000000 ) ) ;
#7774=VERTEX_POINT ( 'NONE', #8323 ) ;
#7776=ORIENTED_EDGE ( 'NONE', *, *, #3611, .T. ) ;
#7777=ORIENTED_EDGE ( 'NONE', *, *, #8597, .T. ) ;
#7778=CARTESIAN_POINT ( 'NONE',  ( -2.293506896408097795, 147.5696653505793279, -25.00000000000000355 ) ) ;
#7780=ORIENTED_EDGE ( 'NONE', *, *, #31, .T. ) ;
#7787=ORIENTED_EDGE ( 'NONE', *, *, #8696, .F. ) ;
#7789=ORIENTED_EDGE ( 'NONE', *, *, #3594, .T. ) ;
#7798=ORIENTED_EDGE ( 'NONE', *, *, #1009, .T. ) ;
#7799=CARTESIAN_POINT ( 'NONE',  ( -23.15769640663940976, -117.1457019118819005, 49.99999999999997868 ) ) ;
#7800=CARTESIAN_POINT ( 'NONE',  ( 80.08610854271792334, 54.73418909528891874, 30.00000000000000355 ) ) ;
#7801=AXIS2_PLACEMENT_3D ( 'NONE', #4901, #43, #9960 ) ;
#7802=DIRECTION ( 'NONE',  ( -1.000000000000000000, 0.000000000000000000, -8.379529552680125332E-16 ) ) ;
#7803=CYLINDRICAL_SURFACE ( 'NONE', #4275, 7.500000000000000000 ) ;
#7804=EDGE_CURVE ( 'NONE', #8577, #8659, #3503, .T. ) ;
#7805=ADVANCED_FACE ( 'NONE', ( #9772 ), #8512, .F. ) ;
#7807=DIRECTION ( 'NONE',  ( 0.000000000000000000, -1.000000000000000000, 0.000000000000000000 ) ) ;
#7808=ORIENTED_EDGE ( 'NONE', *, *, #1687, .T. ) ;
#7809=CARTESIAN_POINT ( 'NONE',  ( -27.15769640663939555, -133.1457019118818721, -27.15769640663944173 ) ) ;
#7817=DIRECTION ( 'NONE',  ( 1.000000000000000000, 0.000000000000000000, 0.000000000000000000 ) ) ;
#7819=EDGE_LOOP ( 'NONE', ( #2181, #1996, #6666, #7039 ) ) ;
#7820=DIRECTION ( 'NONE',  ( -0.000000000000000000, 1.000000000000000000, -0.000000000000000000 ) ) ;
#7823=ORIENTED_EDGE ( 'NONE', *, *, #4238, .F. ) ;
#7825=DIRECTION ( 'NONE',  ( -1.277197683604454965E-16, 1.000000000000000000, -0.000000000000000000 ) ) ;
#7827=ORIENTED_EDGE ( 'NONE', *, *, #8411, .T. ) ;
#7828=CARTESIAN_POINT ( 'NONE',  ( -20.14472382240650816, -141.8229441850657508, 25.87097612368018673 ) ) ;
#7829=CARTESIAN_POINT ( 'NONE',  ( -23.15769640663937423, -117.1457019118819005, -48.00000000000002132 ) ) ;
#7833=DIRECTION ( 'NONE',  ( 0.000000000000000000, 0.000000000000000000, -1.000000000000000000 ) ) ;
#7834=AXIS2_PLACEMENT_3D ( 'NONE', #8285, #6692, #9133 ) ;
#7835=FACE_BOUND ( 'NONE', #4917, .T. ) ;
#7839=ORIENTED_EDGE ( 'NONE', *, *, #4462, .F. ) ;
#7840=CARTESIAN_POINT ( 'NONE',  ( 27.15769640663938489, -117.1457019118819005, -23.15769640663940976 ) ) ;
#7842=ORIENTED_EDGE ( 'NONE', *, *, #6377, .F. ) ;
#7844=DIRECTION ( 'NONE',  ( 0.000000000000000000, 0.000000000000000000, -1.000000000000000000 ) ) ;
#7845=CARTESIAN_POINT ( 'NONE',  ( 37.22511195853868315, -116.3672949040187063, 25.00000000000000000 ) ) ;
#7846=CARTESIAN_POINT ( 'NONE',  ( -23.15769640663937423, -135.1457019118818721, -48.00000000000002132 ) ) ;
#7848=VERTEX_POINT ( 'NONE', #4976 ) ;
#7850=EDGE_LOOP ( 'NONE', ( #5147, #6558, #2105, #9711 ) ) ;
#7851=AXIS2_PLACEMENT_3D ( 'NONE', #589, #6306, #7116 ) ;
#7852=ADVANCED_FACE ( 'NONE', ( #8478 ), #2862, .T. ) ;
#7854=ORIENTED_EDGE ( 'NONE', *, *, #4631, .F. ) ;
#7855=DIRECTION ( 'NONE',  ( -0.000000000000000000, -0.000000000000000000, -1.000000000000000000 ) ) ;
#7861=CARTESIAN_POINT ( 'NONE',  ( -23.15769640663937423, -117.1457019118819005, -48.00000000000002132 ) ) ;
#7864=TOROIDAL_SURFACE ( 'NONE', #2285, 26.75575292317714471, 5.000000000000000000 ) ;
#7865=ADVANCED_FACE ( 'NONE', ( #3665 ), #6145, .F. ) ;
#7869=CIRCLE ( 'NONE', #3467, 3.297986701801175258 ) ;
#7871=FACE_OUTER_BOUND ( 'NONE', #9211, .T. ) ;
#7872=CARTESIAN_POINT ( 'NONE',  ( 37.22511195853868315, -116.3672949040187063, 25.00000000000000000 ) ) ;
#7873=VERTEX_POINT ( 'NONE', #9386 ) ;
#7874=CIRCLE ( 'NONE', #2452, 3.999999999999996447 ) ;
#7877=ORIENTED_EDGE ( 'NONE', *, *, #3926, .F. ) ;
#7878=ADVANCED_FACE ( 'NONE', ( #1958 ), #8588, .F. ) ;
#7885=PLANE ( 'NONE',  #7152 ) ;
#7886=FACE_OUTER_BOUND ( 'NONE', #6335, .T. ) ;
#7887=DIRECTION ( 'NONE',  ( -0.000000000000000000, 1.000000000000000000, -0.000000000000000000 ) ) ;
#7888=CARTESIAN_POINT ( 'NONE',  ( -27.15769640663940976, -115.1457019118818863, 27.15769640663938489 ) ) ;
#7890=FACE_BOUND ( 'NONE', #2657, .T. ) ;
#7893=VECTOR ( 'NONE', #3267, 1000.000000000000000 ) ;
#7894=VERTEX_POINT ( 'NONE', #1330 ) ;
#7895=CARTESIAN_POINT ( 'NONE',  ( -27.15769640663939555, -135.1457019118818721, -27.15769640663944173 ) ) ;
#7897=ORIENTED_EDGE ( 'NONE', *, *, #3140, .T. ) ;
#7898=DIRECTION ( 'NONE',  ( 0.000000000000000000, 0.000000000000000000, 1.000000000000000000 ) ) ;
#7899=DIRECTION ( 'NONE',  ( 1.000000000000000000, 0.000000000000000000, 0.000000000000000000 ) ) ;
#7900=AXIS2_PLACEMENT_3D ( 'NONE', #3089, #6104, #7919 ) ;
#7902=EDGE_CURVE ( 'NONE', #939, #3699, #9225, .T. ) ;
#7904=B_SPLINE_CURVE_WITH_KNOTS ( 'NONE', 3,
 ( #1595, #8055, #5516, #4036, #10353, #1499, #3034, #10401, #10453, #2978 ),
 .UNSPECIFIED., .F., .F.,
 ( 4, 2, 2, 2, 4 ),
 ( -8.944271910604867948E-06, 0.001019331502940706933, 0.002047607277792018454, 0.003075883052643329976, 0.004104158827494642364 ),
 .UNSPECIFIED. ) ;
#7906=ORIENTED_EDGE ( 'NONE', *, *, #8580, .T. ) ;
#7907=VECTOR ( 'NONE', #7203, 1000.000000000000000 ) ;
#7909=( GEOMETRIC_REPRESENTATION_CONTEXT ( 3 ) GLOBAL_UNCERTAINTY_ASSIGNED_CONTEXT ( ( #4204 ) ) GLOBAL_UNIT_ASSIGNED_CONTEXT ( ( #520, #3110, #1527 ) ) REPRESENTATION_CONTEXT ( 'NONE', 'WORKASPACE' ) );
#7914=CIRCLE ( 'NONE', #9085, 2.000000000000001776 ) ;
#7919=DIRECTION ( 'NONE',  ( 0.000000000000000000, -0.000000000000000000, -1.000000000000000000 ) ) ;
#7920=ORIENTED_EDGE ( 'NONE', *, *, #5288, .T. ) ;
#7924=DIRECTION ( 'NONE',  ( 0.000000000000000000, 1.000000000000000000, 0.000000000000000000 ) ) ;
#7925=VECTOR ( 'NONE', #1342, 1000.000000000000000 ) ;
#7930=VERTEX_POINT ( 'NONE', #482 ) ;
#7935=VERTEX_POINT ( 'NONE', #1115 ) ;
#7937=ORIENTED_EDGE ( 'NONE', *, *, #4742, .T. ) ;
#7939=DIRECTION ( 'NONE',  ( 1.000000000000000000, 0.000000000000000000, 8.379529552680124346E-16 ) ) ;
#7942=EDGE_CURVE ( 'NONE', #8369, #4089, #10044, .T. ) ;
#7944=EDGE_CURVE ( 'NONE', #939, #9477, #7325, .T. ) ;
#7945=LINE ( 'NONE', #5553, #4245 ) ;
#7946=VECTOR ( 'NONE', #3372, 1000.000000000000000 ) ;
#7949=VERTEX_POINT ( 'NONE', #7634 ) ;
#7953=VECTOR ( 'NONE', #8308, 1000.000000000000000 ) ;
#7957=DIRECTION ( 'NONE',  ( 1.000000000000000000, 0.000000000000000000, 0.000000000000000000 ) ) ;
#7958=ORIENTED_EDGE ( 'NONE', *, *, #500, .F. ) ;
#7961=PLANE ( 'NONE',  #9102 ) ;
#7962=CARTESIAN_POINT ( 'NONE',  ( -23.15769640663937423, -133.1457019118818721, -48.00000000000002132 ) ) ;
#7963=DIRECTION ( 'NONE',  ( 9.776117811460147207E-16, -0.000000000000000000, -1.000000000000000000 ) ) ;
#7969=ORIENTED_EDGE ( 'NONE', *, *, #5714, .F. ) ;
#7970=AXIS2_PLACEMENT_3D ( 'NONE', #7679, #5286, #2006 ) ;
#7971=CARTESIAN_POINT ( 'NONE',  ( -25.15769640663940265, -115.1457019118818863, -3.513494341946491635E-15 ) ) ;
#7972=B_SPLINE_CURVE_WITH_KNOTS ( 'NONE', 3,
 ( #3134, #9667, #6212, #8008, #2386, #5620, #3893, #2294, #9454, #5415 ),
 .UNSPECIFIED., .F., .F.,
 ( 4, 2, 2, 2, 4 ),
 ( 0.000000000000000000, 0.001023740819106960624, 0.002047481638213921248, 0.003071222457320881873, 0.004094963276427842497 ),
 .UNSPECIFIED. ) ;
#7973=CARTESIAN_POINT ( 'NONE',  ( 26.27514770175546843, -135.1457019118818721, -50.00000000000001421 ) ) ;
#7980=DIRECTION ( 'NONE',  ( -1.000000000000000000, 0.000000000000000000, 0.000000000000000000 ) ) ;
#7982=ORIENTED_EDGE ( 'NONE', *, *, #7347, .T. ) ;
#7983=AXIS2_PLACEMENT_3D ( 'NONE', #1991, #3582, #2887 ) ;
#7985=CARTESIAN_POINT ( 'NONE',  ( 53.40242741783141156, 147.5696653505793279, 25.00000000000000000 ) ) ;
#7986=FACE_OUTER_BOUND ( 'NONE', #8312, .T. ) ;
#7993=EDGE_CURVE ( 'NONE', #898, #869, #5457, .T. ) ;
#7996=CARTESIAN_POINT ( 'NONE',  ( 37.22511195853868315, -116.3672949040186779, -25.00000000000000355 ) ) ;
#7997=CIRCLE ( 'NONE', #6313, 1.999999999999998224 ) ;
#7999=CARTESIAN_POINT ( 'NONE',  ( 37.22511195853869026, -145.1457019118819005, -30.00000000000000355 ) ) ;
#8000=DIRECTION ( 'NONE',  ( -0.000000000000000000, -1.000000000000000000, -0.000000000000000000 ) ) ;
#8001=LINE ( 'NONE', #5612, #9577 ) ;
#8002=EDGE_LOOP ( 'NONE', ( #8301, #1524, #4485, #6686 ) ) ;
#8003=ORIENTED_EDGE ( 'NONE', *, *, #1177, .F. ) ;
#8004=AXIS2_PLACEMENT_3D ( 'NONE', #8276, #3447, #7477 ) ;
#8008=CARTESIAN_POINT ( 'NONE',  ( 25.28852788137212926, -134.8487249201535008, 49.99999999999997868 ) ) ;
#8009=DIRECTION ( 'NONE',  ( 1.000000000000000000, 0.000000000000000000, 6.982941293900105430E-16 ) ) ;
#8013=ORIENTED_EDGE ( 'NONE', *, *, #10202, .T. ) ;
#8016=ORIENTED_EDGE ( 'NONE', *, *, #2562, .T. ) ;
#8019=CARTESIAN_POINT ( 'NONE',  ( 59.99999999999997868, -145.1457019118819005, 30.00000000000000355 ) ) ;
#8021=CARTESIAN_POINT ( 'NONE',  ( 37.39675911933730390, -134.9593434439503312, -26.30486341150395901 ) ) ;
#8022=CIRCLE ( 'NONE', #10411, 3.297986701801175258 ) ;
#8023=ORIENTED_EDGE ( 'NONE', *, *, #80, .T. ) ;
#8028=CARTESIAN_POINT ( 'NONE',  ( 6.756858349438872757, 146.7073643690755773, 30.00000000000000355 ) ) ;
#8029=ORIENTED_EDGE ( 'NONE', *, *, #2562, .F. ) ;
#8030=CIRCLE ( 'NONE', #1941, 31.75575292317714471 ) ;
#8033=DIRECTION ( 'NONE',  ( -0.000000000000000000, 1.000000000000000000, -0.000000000000000000 ) ) ;
#8034=CARTESIAN_POINT ( 'NONE',  ( 27.15769640663938489, -135.1457019118818721, -27.15769640663940976 ) ) ;
#8035=FACE_BOUND ( 'NONE', #6602, .T. ) ;
#8037=ADVANCED_FACE ( 'NONE', ( #9608 ), #2177, .F. ) ;
#8043=LINE ( 'NONE', #5019, #3082 ) ;
#8045=DIRECTION ( 'NONE',  ( 0.000000000000000000, 0.000000000000000000, 1.000000000000000000 ) ) ;
#8048=VERTEX_POINT ( 'NONE', #5506 ) ;
#8051=VECTOR ( 'NONE', #918, 1000.000000000000000 ) ;
#8053=CIRCLE ( 'NONE', #5182, 4.000000000000000000 ) ;
#8055=CARTESIAN_POINT ( 'NONE',  ( -50.00000000000001421, -133.3880685334790144, -23.40006363392675937 ) ) ;
#8061=EDGE_CURVE ( 'NONE', #2182, #826, #3224, .T. ) ;
#8065=ADVANCED_FACE ( 'NONE', ( #643 ), #4759, .F. ) ;
#8066=ORIENTED_EDGE ( 'NONE', *, *, #994, .T. ) ;
#8070=VERTEX_POINT ( 'NONE', #7845 ) ;
#8072=AXIS2_PLACEMENT_3D ( 'NONE', #6495, #9741, #2632 ) ;
#8073=DIRECTION ( 'NONE',  ( -0.000000000000000000, -0.000000000000000000, -1.000000000000000000 ) ) ;
#8075=DIRECTION ( 'NONE',  ( 1.000000000000000000, 0.000000000000000000, 0.000000000000000000 ) ) ;
#8076=AXIS2_PLACEMENT_3D ( 'NONE', #505, #3737, #6968 ) ;
#8077=EDGE_CURVE ( 'NONE', #2596, #2698, #3882, .T. ) ;
#8089=LINE ( 'NONE', #1679, #8304 ) ;
#8090=CARTESIAN_POINT ( 'NONE',  ( 99.80027788547053547, -145.1457019118819005, -27.92893218813452094 ) ) ;
#8091=AXIS2_PLACEMENT_3D ( 'NONE', #7055, #10291, #1433 ) ;
#8094=AXIS2_PLACEMENT_3D ( 'NONE', #10374, #9586, #4699 ) ;
#8095=VERTEX_POINT ( 'NONE', #4028 ) ;
#8097=DIRECTION ( 'NONE',  ( 1.000000000000000000, 0.000000000000000000, 1.396588258780020149E-16 ) ) ;
#8099=LINE ( 'NONE', #163, #3957 ) ;
#8100=LINE ( 'NONE', #7310, #1446 ) ;
#8101=CARTESIAN_POINT ( 'NONE',  ( 77.30044127146538813, 73.68369600860394542, -12.50000000000000000 ) ) ;
#8103=ORIENTED_EDGE ( 'NONE', *, *, #3524, .F. ) ;
#8106=ORIENTED_EDGE ( 'NONE', *, *, #8061, .T. ) ;
#8109=EDGE_CURVE ( 'NONE', #3359, #5589, #4073, .T. ) ;
#8114=VERTEX_POINT ( 'NONE', #4183 ) ;
#8115=PLANE ( 'NONE',  #9936 ) ;
#8116=ORIENTED_EDGE ( 'NONE', *, *, #5096, .F. ) ;
#8117=CARTESIAN_POINT ( 'NONE',  ( -2.293506896408097795, 37.08684478514406635, -24.99999999999998934 ) ) ;
#8118=ORIENTED_EDGE ( 'NONE', *, *, #1262, .F. ) ;
#8123=EDGE_CURVE ( 'NONE', #4400, #9740, #8099, .T. ) ;
#8125=DIRECTION ( 'NONE',  ( 1.000000000000000000, -8.585830317548973933E-16, 0.000000000000000000 ) ) ;
#8127=ORIENTED_EDGE ( 'NONE', *, *, #9639, .T. ) ;
#8128=FACE_OUTER_BOUND ( 'NONE', #1030, .T. ) ;
#8130=ORIENTED_EDGE ( 'NONE', *, *, #5069, .F. ) ;
#8136=DIRECTION ( 'NONE',  ( -1.000000000000000000, -0.000000000000000000, 0.000000000000000000 ) ) ;
#8138=DIRECTION ( 'NONE',  ( 0.000000000000000000, 0.000000000000000000, -1.000000000000000000 ) ) ;
#8140=EDGE_LOOP ( 'NONE', ( #8596, #7760, #2837, #111 ) ) ;
#8141=AXIS2_PLACEMENT_3D ( 'NONE', #5213, #348, #5312 ) ;
#8148=CARTESIAN_POINT ( 'NONE',  ( 14.70649310359190309, 80.56966535057935630, -16.00000000000000711 ) ) ;
#8152=DIRECTION ( 'NONE',  ( -0.000000000000000000, 1.000000000000000000, 0.000000000000000000 ) ) ;
#8153=AXIS2_PLACEMENT_3D ( 'NONE', #1274, #1169, #6948 ) ;
#8155=EDGE_CURVE ( 'NONE', #6555, #4407, #7340, .T. ) ;
#8159=EDGE_LOOP ( 'NONE', ( #6221, #4913, #873, #6281 ) ) ;
#8160=AXIS2_PLACEMENT_3D ( 'NONE', #5539, #563, #2358 ) ;
#8162=DIRECTION ( 'NONE',  ( -0.000000000000000000, 1.000000000000000000, -0.000000000000000000 ) ) ;
#8165=ORIENTED_EDGE ( 'NONE', *, *, #9849, .T. ) ;
#8167=VECTOR ( 'NONE', #7493, 1000.000000000000000 ) ;
#8169=CIRCLE ( 'NONE', #1058, 10.00000000000000178 ) ;
#8172=ORIENTED_EDGE ( 'NONE', *, *, #9829, .F. ) ;
#8173=ORIENTED_EDGE ( 'NONE', *, *, #3139, .F. ) ;
#8175=FACE_OUTER_BOUND ( 'NONE', #7550, .T. ) ;
#8176=AXIS2_PLACEMENT_3D ( 'NONE', #6895, #2015, #2119 ) ;
#8177=CARTESIAN_POINT ( 'NONE',  ( 59.99999999999999289, 52.77167129626698028, -30.00000000000000355 ) ) ;
#8178=DIRECTION ( 'NONE',  ( -0.7367503238654704578, -0.6761648913424330720, 0.000000000000000000 ) ) ;
#8180=DIRECTION ( 'NONE',  ( 0.000000000000000000, 0.000000000000000000, 1.000000000000000000 ) ) ;
#8181=ORIENTED_EDGE ( 'NONE', *, *, #2371, .T. ) ;
#8182=CARTESIAN_POINT ( 'NONE',  ( 85.07264007511442117, 55.10093597859600578, -24.99999999999998934 ) ) ;
#8184=CIRCLE ( 'NONE', #406, 3.297986701801175258 ) ;
#8185=EDGE_CURVE ( 'NONE', #2154, #8341, #5811, .T. ) ;
#8190=ORIENTED_EDGE ( 'NONE', *, *, #1584, .T. ) ;
#8192=DIRECTION ( 'NONE',  ( -0.000000000000000000, 1.000000000000000000, -0.000000000000000000 ) ) ;
#8201=CIRCLE ( 'NONE', #5148, 2.000000000000001776 ) ;
#8202=DIRECTION ( 'NONE',  ( 1.000000000000000000, 0.000000000000000000, 0.000000000000000000 ) ) ;
#8203=ORIENTED_EDGE ( 'NONE', *, *, #128, .F. ) ;
#8204=LINE ( 'NONE', #837, #7259 ) ;
#8205=FACE_OUTER_BOUND ( 'NONE', #8749, .T. ) ;
#8209=FACE_OUTER_BOUND ( 'NONE', #9937, .T. ) ;
#8210=VECTOR ( 'NONE', #7957, 1000.000000000000000 ) ;
#8211=DIRECTION ( 'NONE',  ( 1.000000000000000000, 0.000000000000000000, 0.000000000000000000 ) ) ;
#8212=AXIS2_PLACEMENT_3D ( 'NONE', #9484, #8627, #7833 ) ;
#8213=ORIENTED_EDGE ( 'NONE', *, *, #8109, .F. ) ;
#8214=ORIENTED_EDGE ( 'NONE', *, *, #8317, .T. ) ;
#8215=ORIENTED_EDGE ( 'NONE', *, *, #5833, .T. ) ;
#8222=ORIENTED_EDGE ( 'NONE', *, *, #5767, .T. ) ;
#8223=DIRECTION ( 'NONE',  ( 0.07334937666141774781, -0.9973063064792991872, 2.035854170285226689E-16 ) ) ;
#8225=ORIENTED_EDGE ( 'NONE', *, *, #4311, .F. ) ;
#8227=EDGE_LOOP ( 'NONE', ( #7431, #349, #6610, #8003, #8269, #6384 ) ) ;
#8234=AXIS2_PLACEMENT_3D ( 'NONE', #1346, #7807, #548 ) ;
#8235=DIRECTION ( 'NONE',  ( -0.000000000000000000, -0.000000000000000000, -1.000000000000000000 ) ) ;
#8238=LINE ( 'NONE', #1614, #4948 ) ;
#8239=VECTOR ( 'NONE', #7825, 1000.000000000000000 ) ;
#8242=CARTESIAN_POINT ( 'NONE',  ( -23.40006363390418187, -133.3880685335015812, 49.99999999999997158 ) ) ;
#8248=DIRECTION ( 'NONE',  ( 0.000000000000000000, 0.000000000000000000, 1.000000000000000000 ) ) ;
#8249=CYLINDRICAL_SURFACE ( 'NONE', #7801, 5.000000000000000888 ) ;
#8251=CARTESIAN_POINT ( 'NONE',  ( 37.22511195853866894, 17.84145331825996195, 25.00000000000000000 ) ) ;
#8253=ORIENTED_EDGE ( 'NONE', *, *, #10086, .T. ) ;
#8261=EDGE_CURVE ( 'NONE', #3742, #3983, #9002, .T. ) ;
#8265=CIRCLE ( 'NONE', #2005, 2.000000000000001776 ) ;
#8266=CARTESIAN_POINT ( 'NONE',  ( 39.99999999999997158, -135.1457019118818721, 43.99999999999997158 ) ) ;
#8268=AXIS2_PLACEMENT_3D ( 'NONE', #1416, #8934, #6599 ) ;
#8269=ORIENTED_EDGE ( 'NONE', *, *, #8411, .F. ) ;
#8270=AXIS2_PLACEMENT_3D ( 'NONE', #2587, #208, #9916 ) ;
#8271=ORIENTED_EDGE ( 'NONE', *, *, #10145, .F. ) ;
#8272=CARTESIAN_POINT ( 'NONE',  ( -16.29350689640809691, -140.1746510883711778, 27.01918567566963247 ) ) ;
#8274=EDGE_CURVE ( 'NONE', #9740, #2723, #2765, .T. ) ;
#8276=CARTESIAN_POINT ( 'NONE',  ( 4.856471286862176662, 145.0444252872335937, 30.00000000000000355 ) ) ;
#8282=CARTESIAN_POINT ( 'NONE',  ( 37.22759939293836595, -115.1457019118818863, -25.15769640663939910 ) ) ;
#8283=CARTESIAN_POINT ( 'NONE',  ( -23.15769640663937423, -115.1457019118818863, -48.00000000000002132 ) ) ;
#8284=CARTESIAN_POINT ( 'NONE',  ( 25.15769640663940265, -133.1457019118818721, -48.00000000000002132 ) ) ;
#8285=CARTESIAN_POINT ( 'NONE',  ( 23.15769640663936713, -117.1457019118819005, 47.99999999999997868 ) ) ;
#8286=AXIS2_PLACEMENT_3D ( 'NONE', #3810, #627, #5493 ) ;
#8289=DIRECTION ( 'NONE',  ( 1.000000000000000000, 0.000000000000000000, 0.000000000000000000 ) ) ;
#8292=DIRECTION ( 'NONE',  ( 0.000000000000000000, 0.000000000000000000, 1.000000000000000000 ) ) ;
#8294=VERTEX_POINT ( 'NONE', #2793 ) ;
#8295=CARTESIAN_POINT ( 'NONE',  ( 99.80027788547049283, -145.1457019118818721, 27.92893218813452094 ) ) ;
#8296=CARTESIAN_POINT ( 'NONE',  ( -23.76520584195948516, -145.1457019118819005, -97.78965767959371647 ) ) ;
#8297=PLANE ( 'NONE',  #6860 ) ;
#8300=EDGE_CURVE ( 'NONE', #172, #8048, #5136, .T. ) ;
#8301=ORIENTED_EDGE ( 'NONE', *, *, #8711, .F. ) ;
#8303=B_SPLINE_CURVE_WITH_KNOTS ( 'NONE', 3,
 ( #7872, #4691, #10416, #9411 ),
 .UNSPECIFIED., .F., .F.,
 ( 4, 4 ),
 ( 1.430489624538199204E-17, 0.0007942240325546766778 ),
 .UNSPECIFIED. ) ;
#8304=VECTOR ( 'NONE', #9046, 1000.000000000000000 ) ;
#8308=DIRECTION ( 'NONE',  ( 0.000000000000000000, 0.000000000000000000, 1.000000000000000000 ) ) ;
#8310=FACE_OUTER_BOUND ( 'NONE', #6598, .T. ) ;
#8312=EDGE_LOOP ( 'NONE', ( #6229, #6297, #1579, #2865 ) ) ;
#8313=VECTOR ( 'NONE', #2980, 1000.000000000000000 ) ;
#8315=EDGE_CURVE ( 'NONE', #7894, #8878, #7729, .T. ) ;
#8316=ORIENTED_EDGE ( 'NONE', *, *, #905, .T. ) ;
#8317=EDGE_CURVE ( 'NONE', #8095, #1304, #8521, .T. ) ;
#8323=CARTESIAN_POINT ( 'NONE',  ( 17.97972049165455388, 42.08684478514406635, -30.00000000000000355 ) ) ;
#8327=ORIENTED_EDGE ( 'NONE', *, *, #6900, .F. ) ;
#8330=AXIS2_PLACEMENT_3D ( 'NONE', #6746, #4936, #8337 ) ;
#8332=TOROIDAL_SURFACE ( 'NONE', #4768, 4.000000000000000000, 2.000000000000000000 ) ;
#8333=EDGE_LOOP ( 'NONE', ( #7119, #3048, #243, #2085 ) ) ;
#8336=DIRECTION ( 'NONE',  ( 0.000000000000000000, -1.000000000000000000, 0.000000000000000000 ) ) ;
#8337=DIRECTION ( 'NONE',  ( -0.7525569905852205199, -0.6585271261848794078, 0.000000000000000000 ) ) ;
#8341=VERTEX_POINT ( 'NONE', #8573 ) ;
#8348=CARTESIAN_POINT ( 'NONE',  ( -25.15769640663940621, -117.1457019118819005, 25.15769640663938134 ) ) ;
#8349=CARTESIAN_POINT ( 'NONE',  ( 37.31363630694986711, -134.7663435696292709, 25.95623500213750035 ) ) ;
#8352=CARTESIAN_POINT ( 'NONE',  ( -16.29350689640809691, -140.1746510883711778, -30.31717237747080773 ) ) ;
#8356=ORIENTED_EDGE ( 'NONE', *, *, #4194, .F. ) ;
#8358=AXIS2_PLACEMENT_3D ( 'NONE', #628, #726, #3059 ) ;
#8363=DIRECTION ( 'NONE',  ( 0.000000000000000000, 1.000000000000000000, 0.000000000000000000 ) ) ;
#8364=DIRECTION ( 'NONE',  ( 0.000000000000000000, 0.000000000000000000, 1.000000000000000000 ) ) ;
#8365=EDGE_CURVE ( 'NONE', #5357, #6846, #9889, .T. ) ;
#8369=VERTEX_POINT ( 'NONE', #9216 ) ;
#8372=PLANE ( 'NONE',  #5040 ) ;
#8374=AXIS2_PLACEMENT_3D ( 'NONE', #6408, #9555, #1639 ) ;
#8377=FACE_OUTER_BOUND ( 'NONE', #8483, .T. ) ;
#8378=EDGE_CURVE ( 'NONE', #4419, #415, #8860, .T. ) ;
#8383=DIRECTION ( 'NONE',  ( 0.000000000000000000, -1.000000000000000000, 0.000000000000000000 ) ) ;
#8384=ORIENTED_EDGE ( 'NONE', *, *, #9190, .T. ) ;
#8387=DIRECTION ( 'NONE',  ( 0.000000000000000000, 0.000000000000000000, 1.000000000000000000 ) ) ;
#8391=ADVANCED_FACE ( 'NONE', ( #421 ), #10396, .F. ) ;
#8395=ORIENTED_EDGE ( 'NONE', *, *, #9165, .T. ) ;
#8396=DIRECTION ( 'NONE',  ( -0.000000000000000000, 1.000000000000000000, -0.000000000000000000 ) ) ;
#8398=TOROIDAL_SURFACE ( 'NONE', #2305, 24.24539146688411506, 5.000000000000000000 ) ;
#8399=DIRECTION ( 'NONE',  ( 0.000000000000000000, 0.000000000000000000, 1.000000000000000000 ) ) ;
#8400=ORIENTED_EDGE ( 'NONE', *, *, #3566, .F. ) ;
#8401=AXIS2_PLACEMENT_3D ( 'NONE', #7861, #5418, #9570 ) ;
#8403=CARTESIAN_POINT ( 'NONE',  ( -40.00000000000001421, -135.1457019118818721, -50.00000000000002132 ) ) ;
#8405=CARTESIAN_POINT ( 'NONE',  ( 14.70649310359190309, 80.56966535057935630, 24.00000000000000711 ) ) ;
#8411=EDGE_CURVE ( 'NONE', #2186, #9448, #8184, .T. ) ;
#8413=CARTESIAN_POINT ( 'NONE',  ( -16.29350689640809691, -140.1746510883711778, 0.000000000000000000 ) ) ;
#8414=ORIENTED_EDGE ( 'NONE', *, *, #10135, .F. ) ;
#8415=DIRECTION ( 'NONE',  ( -0.9973063064792988541, -0.07334937666141910784, 0.000000000000000000 ) ) ;
#8416=FACE_OUTER_BOUND ( 'NONE', #2998, .T. ) ;
#8418=CARTESIAN_POINT ( 'NONE',  ( -16.29350689640809691, -140.1746510883711778, -27.01918567566963247 ) ) ;
#8424=ADVANCED_FACE ( 'NONE', ( #5130 ), #8523, .F. ) ;
#8426=CARTESIAN_POINT ( 'NONE',  ( -40.00000000000001421, -135.1457019118818721, -36.00000000000002842 ) ) ;
#8430=DIRECTION ( 'NONE',  ( 0.000000000000000000, 0.000000000000000000, -1.000000000000000000 ) ) ;
#8432=DIRECTION ( 'NONE',  ( -1.000000000000000000, 0.000000000000000000, 0.000000000000000000 ) ) ;
#8433=EDGE_LOOP ( 'NONE', ( #4043, #5801, #10057, #8473 ) ) ;
#8434=DIRECTION ( 'NONE',  ( -1.000000000000000000, -0.000000000000000000, -0.000000000000000000 ) ) ;
#8437=ORIENTED_EDGE ( 'NONE', *, *, #5270, .T. ) ;
#8438=DIRECTION ( 'NONE',  ( 0.000000000000000000, 0.000000000000000000, -1.000000000000000000 ) ) ;
#8440=CARTESIAN_POINT ( 'NONE',  ( -23.15769640663937423, -117.1457019118819005, -48.00000000000002132 ) ) ;
#8441=CARTESIAN_POINT ( 'NONE',  ( -16.29350689640809691, -186.9457019118818835, 0.000000000000000000 ) ) ;
#8444=VECTOR ( 'NONE', #9793, 1000.000000000000000 ) ;
#8446=EDGE_CURVE ( 'NONE', #2463, #8659, #3622, .T. ) ;
#8447=VERTEX_POINT ( 'NONE', #5390 ) ;
#8454=CARTESIAN_POINT ( 'NONE',  ( 37.36104957496461765, -134.9117008620985985, 26.18446763346474171 ) ) ;
#8456=CYLINDRICAL_SURFACE ( 'NONE', #5438, 4.000000000000000000 ) ;
#8457=ORIENTED_EDGE ( 'NONE', *, *, #9487, .T. ) ;
#8458=LINE ( 'NONE', #462, #2249 ) ;
#8459=ORIENTED_EDGE ( 'NONE', *, *, #1774, .F. ) ;
#8461=ORIENTED_EDGE ( 'NONE', *, *, #8903, .T. ) ;
#8463=LINE ( 'NONE', #4588, #8239 ) ;
#8466=CARTESIAN_POINT ( 'NONE',  ( 94.81374635307400922, -145.5124487951889876, -25.00000000000000355 ) ) ;
#8469=CARTESIAN_POINT ( 'NONE',  ( -23.15769640663940976, -117.1457019118819005, 47.99999999999997868 ) ) ;
#8470=CARTESIAN_POINT ( 'NONE',  ( -25.15769640663940976, -117.1457019118819005, 47.99999999999997868 ) ) ;
#8473=ORIENTED_EDGE ( 'NONE', *, *, #1959, .T. ) ;
#8478=FACE_OUTER_BOUND ( 'NONE', #1916, .T. ) ;
#8479=EDGE_CURVE ( 'NONE', #4826, #8668, #4134, .T. ) ;
#8480=FACE_OUTER_BOUND ( 'NONE', #2900, .T. ) ;
#8482=ORIENTED_EDGE ( 'NONE', *, *, #10070, .T. ) ;
#8483=EDGE_LOOP ( 'NONE', ( #9764, #5091, #9805, #7024 ) ) ;
#8484=DIRECTION ( 'NONE',  ( 8.659560562356134638E-17, 0.7071067811864494290, -0.7071067811866454944 ) ) ;
#8486=ORIENTED_EDGE ( 'NONE', *, *, #10398, .F. ) ;
#8487=VECTOR ( 'NONE', #8490, 1000.000000000000000 ) ;
#8488=ORIENTED_EDGE ( 'NONE', *, *, #8967, .T. ) ;
#8490=DIRECTION ( 'NONE',  ( -1.396588258780021135E-16, -0.000000000000000000, 1.000000000000000000 ) ) ;
#8491=CARTESIAN_POINT ( 'NONE',  ( -48.00000000000002132, -133.1457019118818721, -25.15769640663945950 ) ) ;
#8492=CARTESIAN_POINT ( 'NONE',  ( 1.940506014114293224E-14, -115.1457019118818863, -23.15769640663941331 ) ) ;
#8493=ADVANCED_FACE ( 'NONE', ( #8786 ), #8626, .T. ) ;
#8495=VECTOR ( 'NONE', #9372, 1000.000000000000000 ) ;
#8500=CARTESIAN_POINT ( 'NONE',  ( 99.80027788547049283, -145.1457019118819005, 30.00000000000000355 ) ) ;
#8502=VECTOR ( 'NONE', #5587, 1000.000000000000000 ) ;
#8504=CARTESIAN_POINT ( 'NONE',  ( 37.26943424014034889, -134.4902506524434500, 25.67119517670793627 ) ) ;
#8505=EDGE_CURVE ( 'NONE', #836, #9808, #73, .T. ) ;
#8508=EDGE_CURVE ( 'NONE', #3326, #2357, #6290, .T. ) ;
#8511=CARTESIAN_POINT ( 'NONE',  ( -40.00000000000001421, -135.1707019118818778, -44.00000000000002132 ) ) ;
#8512=CONICAL_SURFACE ( 'NONE', #1576, 4.025000000000000355, 0.7853981633975870569 ) ;
#8515=EDGE_LOOP ( 'NONE', ( #176, #3657, #9149, #6236, #3029, #3819, #7958, #3373, #8116, #4388 ) ) ;
#8516=CARTESIAN_POINT ( 'NONE',  ( 25.15769640663936357, -133.1457019118818721, 27.15769640663938489 ) ) ;
#8518=EDGE_LOOP ( 'NONE', ( #4764, #2611, #3647, #8222 ) ) ;
#8521=CIRCLE ( 'NONE', #574, 2.000000000000001776 ) ;
#8522=DIRECTION ( 'NONE',  ( 0.000000000000000000, -1.000000000000000000, 0.000000000000000000 ) ) ;
#8523=CYLINDRICAL_SURFACE ( 'NONE', #6659, 3.999999999999989786 ) ;
#8525=EDGE_CURVE ( 'NONE', #2815, #2514, #9723, .T. ) ;
#8534=LINE ( 'NONE', #2755, #4378 ) ;
#8536=CARTESIAN_POINT ( 'NONE',  ( -50.00000000000002132, -135.1457019118818721, -6.938893903907231533E-15 ) ) ;
#8540=ORIENTED_EDGE ( 'NONE', *, *, #5919, .F. ) ;
#8544=ORIENTED_EDGE ( 'NONE', *, *, #6276, .T. ) ;
#8545=ORIENTED_EDGE ( 'NONE', *, *, #2682, .T. ) ;
#8547=LINE ( 'NONE', #8600, #8313 ) ;
#8548=AXIS2_PLACEMENT_3D ( 'NONE', #6723, #9974, #2481 ) ;
#8550=DIRECTION ( 'NONE',  ( 0.000000000000000000, 0.000000000000000000, 1.000000000000000000 ) ) ;
#8553=CARTESIAN_POINT ( 'NONE',  ( -40.00000000000002842, -135.1457019118818721, 39.99999999999997868 ) ) ;
#8556=VECTOR ( 'NONE', #6170, 1000.000000000000000 ) ;
#8558=CARTESIAN_POINT ( 'NONE',  ( 27.15769640663938489, -133.1457019118818721, -27.15769640663940976 ) ) ;
#8559=CARTESIAN_POINT ( 'NONE',  ( 14.70649310359190309, 80.56966535057935630, -24.00000000000000711 ) ) ;
#8561=CARTESIAN_POINT ( 'NONE',  ( 27.15769640663938489, -117.1457019118819005, -25.15769640663940621 ) ) ;
#8563=ORIENTED_EDGE ( 'NONE', *, *, #7336, .F. ) ;
#8565=DIRECTION ( 'NONE',  ( -0.000000000000000000, -0.000000000000000000, -1.000000000000000000 ) ) ;
#8566=EDGE_CURVE ( 'NONE', #7848, #4047, #4796, .T. ) ;
#8567=VERTEX_POINT ( 'NONE', #5494 ) ;
#8568=ORIENTED_EDGE ( 'NONE', *, *, #4238, .T. ) ;
#8571=AXIS2_PLACEMENT_3D ( 'NONE', #3188, #8009, #2295 ) ;
#8573=CARTESIAN_POINT ( 'NONE',  ( -23.76520584195948516, -145.1457019118819005, 0.6509338422959615178 ) ) ;
#8577=VERTEX_POINT ( 'NONE', #6185 ) ;
#8580=EDGE_CURVE ( 'NONE', #8605, #9452, #10059, .T. ) ;
#8582=EDGE_CURVE ( 'NONE', #3508, #3785, #5646, .T. ) ;
#8583=VECTOR ( 'NONE', #2576, 1000.000000000000000 ) ;
#8585=FACE_OUTER_BOUND ( 'NONE', #8774, .T. ) ;
#8586=CARTESIAN_POINT ( 'NONE',  ( 0.000000000000000000, 0.000000000000000000, 0.000000000000000000 ) ) ;
#8587=VERTEX_POINT ( 'NONE', #8884 ) ;
#8588=CYLINDRICAL_SURFACE ( 'NONE', #9881, 3.297986701801175258 ) ;
#8590=AXIS2_PLACEMENT_3D ( 'NONE', #4477, #3949, #5678 ) ;
#8593=ORIENTED_EDGE ( 'NONE', *, *, #1843, .T. ) ;
#8596=ORIENTED_EDGE ( 'NONE', *, *, #225, .T. ) ;
#8597=EDGE_CURVE ( 'NONE', #7029, #2154, #9351, .T. ) ;
#8598=EDGE_LOOP ( 'NONE', ( #464, #2881 ) ) ;
#8599=LINE ( 'NONE', #1181, #7925 ) ;
#8600=CARTESIAN_POINT ( 'NONE',  ( 4.856471286862173997, 152.5696653505793279, 25.00000000000000000 ) ) ;
#8603=PLANE ( 'NONE',  #8234 ) ;
#8604=CIRCLE ( 'NONE', #9110, 2.000000000000001776 ) ;
#8605=VERTEX_POINT ( 'NONE', #932 ) ;
#8607=VECTOR ( 'NONE', #9847, 1000.000000000000000 ) ;
#8608=CARTESIAN_POINT ( 'NONE',  ( 2.275687196221499263E-14, -133.1457019118818721, -27.15769640663943107 ) ) ;
#8609=ORIENTED_EDGE ( 'NONE', *, *, #4285, .F. ) ;
#8612=LINE ( 'NONE', #7027, #6848 ) ;
#8613=EDGE_CURVE ( 'NONE', #8605, #8567, #774, .T. ) ;
#8616=CYLINDRICAL_SURFACE ( 'NONE', #2401, 7.500000000000000000 ) ;
#8619=FACE_OUTER_BOUND ( 'NONE', #2973, .T. ) ;
#8626=CYLINDRICAL_SURFACE ( 'NONE', #3118, 5.000000000000000888 ) ;
#8627=DIRECTION ( 'NONE',  ( 0.000000000000000000, -1.000000000000000000, 0.000000000000000000 ) ) ;
#8632=DIRECTION ( 'NONE',  ( 0.000000000000000000, -1.000000000000000000, 0.000000000000000000 ) ) ;
#8639=VERTEX_POINT ( 'NONE', #4016 ) ;
#8643=EDGE_LOOP ( 'NONE', ( #10412, #2011, #6726, #2100 ) ) ;
#8647=DIRECTION ( 'NONE',  ( -0.000000000000000000, 1.000000000000000000, -0.000000000000000000 ) ) ;
#8648=CARTESIAN_POINT ( 'NONE',  ( 99.80027788547049283, -145.1457019118819005, -25.00000000000000355 ) ) ;
#8649=AXIS2_PLACEMENT_3D ( 'NONE', #5183, #523, #1162 ) ;
#8654=EDGE_LOOP ( 'NONE', ( #5125, #280, #7556, #76 ) ) ;
#8656=AXIS2_PLACEMENT_3D ( 'NONE', #4737, #10472, #9413 ) ;
#8658=VERTEX_POINT ( 'NONE', #9852 ) ;
#8659=VERTEX_POINT ( 'NONE', #7247 ) ;
#8661=CARTESIAN_POINT ( 'NONE',  ( 37.59878849545336266, 37.08684478514405214, 12.50000000000000000 ) ) ;
#8664=CARTESIAN_POINT ( 'NONE',  ( 23.15769640663940265, -117.1457019118819005, -50.00000000000002132 ) ) ;
#8666=CARTESIAN_POINT ( 'NONE',  ( 39.99999999999998579, -135.1457019118818721, -50.00000000000002132 ) ) ;
#8668=VERTEX_POINT ( 'NONE', #5804 ) ;
#8669=CIRCLE ( 'NONE', #4434, 2.000000000000001776 ) ;
#8672=ADVANCED_FACE ( 'NONE', ( #986, #150 ), #3264, .F. ) ;
#8673=ORIENTED_EDGE ( 'NONE', *, *, #6324, .T. ) ;
#8674=CARTESIAN_POINT ( 'NONE',  ( -18.34874108452141783, -140.1746510883711778, 29.59847408863694440 ) ) ;
#8675=LINE ( 'NONE', #8729, #3601 ) ;
#8676=PLANE ( 'NONE',  #1010 ) ;
#8677=DIRECTION ( 'NONE',  ( -0.000000000000000000, -0.000000000000000000, 1.000000000000000000 ) ) ;
#8680=DIRECTION ( 'NONE',  ( 1.000000000000000000, 1.748065976125624994E-15, 0.000000000000000000 ) ) ;
#8681=VECTOR ( 'NONE', #8396, 1000.000000000000000 ) ;
#8684=DIRECTION ( 'NONE',  ( -1.000000000000000000, 0.000000000000000000, 0.000000000000000000 ) ) ;
#8688=CARTESIAN_POINT ( 'NONE',  ( -40.00000000000001421, -145.1457019118819005, -50.00000000000002132 ) ) ;
#8695=ORIENTED_EDGE ( 'NONE', *, *, #3139, .T. ) ;
#8696=EDGE_CURVE ( 'NONE', #996, #2723, #3630, .T. ) ;
#8698=ORIENTED_EDGE ( 'NONE', *, *, #4050, .F. ) ;
#8699=EDGE_CURVE ( 'NONE', #5224, #2732, #7692, .T. ) ;
#8700=CARTESIAN_POINT ( 'NONE',  ( -23.15769640663937423, -133.1457019118818721, -50.00000000000002132 ) ) ;
#8701=DIRECTION ( 'NONE',  ( 0.000000000000000000, 0.000000000000000000, -1.000000000000000000 ) ) ;
#8703=EDGE_CURVE ( 'NONE', #1800, #9582, #10232, .T. ) ;
#8707=ORIENTED_EDGE ( 'NONE', *, *, #6866, .T. ) ;
#8708=LINE ( 'NONE', #7021, #4615 ) ;
#8710=EDGE_LOOP ( 'NONE', ( #6424, #5408, #2840, #1724, #9952, #8013 ) ) ;
#8711=EDGE_CURVE ( 'NONE', #4318, #869, #1591, .T. ) ;
#8714=ADVANCED_FACE ( 'NONE', ( #5165 ), #2087, .F. ) ;
#8715=CIRCLE ( 'NONE', #1604, 3.999999999999989786 ) ;
#8716=PLANE ( 'NONE',  #963 ) ;
#8718=DIRECTION ( 'NONE',  ( -1.277197683604454965E-16, 1.000000000000000000, 0.000000000000000000 ) ) ;
#8719=ORIENTED_EDGE ( 'NONE', *, *, #9261, .T. ) ;
#8723=ORIENTED_EDGE ( 'NONE', *, *, #4311, .T. ) ;
#8726=AXIS2_PLACEMENT_3D ( 'NONE', #775, #10431, #3812 ) ;
#8727=ADVANCED_FACE ( 'NONE', ( #6708 ), #1035, .F. ) ;
#8729=CARTESIAN_POINT ( 'NONE',  ( 77.30044127146540234, 73.68369600860394542, 30.00000000000000355 ) ) ;
#8731=CARTESIAN_POINT ( 'NONE',  ( 4.856471286862176662, 145.0444252872335937, -25.00000000000003197 ) ) ;
#8734=PLANE ( 'NONE',  #8989 ) ;
#8736=EDGE_CURVE ( 'NONE', #9477, #1670, #3580, .T. ) ;
#8738=VERTEX_POINT ( 'NONE', #2728 ) ;
#8739=CARTESIAN_POINT ( 'NONE',  ( -23.76520584195948516, -145.1457019118819005, -0.6509338422960262438 ) ) ;
#8740=VECTOR ( 'NONE', #1598, 1000.000000000000000 ) ;
#8742=CARTESIAN_POINT ( 'NONE',  ( -48.00000000000002132, -117.1457019118819005, -6.661338147750942398E-15 ) ) ;
#8749=EDGE_LOOP ( 'NONE', ( #8214, #2517, #10188, #5014 ) ) ;
#8756=FACE_OUTER_BOUND ( 'NONE', #4264, .T. ) ;
#8761=VECTOR ( 'NONE', #9226, 1000.000000000000000 ) ;
#8762=CARTESIAN_POINT ( 'NONE',  ( 0.000000000000000000, -135.1457019118818721, -50.00000000000002132 ) ) ;
#8763=ORIENTED_EDGE ( 'NONE', *, *, #3149, .F. ) ;
#8765=EDGE_CURVE ( 'NONE', #2586, #3286, #10222, .T. ) ;
#8770=AXIS2_PLACEMENT_3D ( 'NONE', #586, #10236, #2174 ) ;
#8771=FACE_OUTER_BOUND ( 'NONE', #1910, .T. ) ;
#8772=CARTESIAN_POINT ( 'NONE',  ( 24.15110854952564168, -134.0910177696405299, -50.00000000000002132 ) ) ;
#8774=EDGE_LOOP ( 'NONE', ( #8922, #8782, #5716, #359, #6013 ) ) ;
#8782=ORIENTED_EDGE ( 'NONE', *, *, #1696, .F. ) ;
#8784=ORIENTED_EDGE ( 'NONE', *, *, #7689, .T. ) ;
#8786=FACE_OUTER_BOUND ( 'NONE', #7063, .T. ) ;
#8787=DIRECTION ( 'NONE',  ( 0.000000000000000000, 0.000000000000000000, 1.000000000000000000 ) ) ;
#8793=LINE ( 'NONE', #48, #6031 ) ;
#8795=CARTESIAN_POINT ( 'NONE',  ( 39.99999999999997158, -145.1457019118819005, 39.99999999999997868 ) ) ;
#8797=EDGE_LOOP ( 'NONE', ( #226, #4751, #5548, #8723 ) ) ;
#8799=DIRECTION ( 'NONE',  ( 1.000000000000000000, 0.000000000000000000, 0.000000000000000000 ) ) ;
#8803=ORIENTED_EDGE ( 'NONE', *, *, #8378, .F. ) ;
#8805=FACE_OUTER_BOUND ( 'NONE', #6487, .T. ) ;
#8806=EDGE_CURVE ( 'NONE', #3545, #3742, #3449, .T. ) ;
#8807=CARTESIAN_POINT ( 'NONE',  ( 39.99999999999997158, -135.1457019118818721, 49.99999999999997868 ) ) ;
#8808=CARTESIAN_POINT ( 'NONE',  ( -25.28852788137214347, -134.8487249201535008, -50.00000000000002132 ) ) ;
#8810=ORIENTED_EDGE ( 'NONE', *, *, #7749, .T. ) ;
#8811=DIRECTION ( 'NONE',  ( 0.000000000000000000, 0.000000000000000000, -1.000000000000000000 ) ) ;
#8813=AXIS2_PLACEMENT_3D ( 'NONE', #3756, #5235, #3602 ) ;
#8814=DIRECTION ( 'NONE',  ( 1.000000000000000000, 0.000000000000000000, 0.000000000000000000 ) ) ;
#8816=ADVANCED_FACE ( 'NONE', ( #10049 ), #4480, .T. ) ;
#8819=ORIENTED_EDGE ( 'NONE', *, *, #3498, .F. ) ;
#8822=ORIENTED_EDGE ( 'NONE', *, *, #7256, .T. ) ;
#8826=CIRCLE ( 'NONE', #1389, 4.000000000000000000 ) ;
#8827=ORIENTED_EDGE ( 'NONE', *, *, #8699, .F. ) ;
#8829=EDGE_CURVE ( 'NONE', #2017, #5655, #7023, .T. ) ;
#8830=DIRECTION ( 'NONE',  ( -1.000000000000000000, 0.000000000000000000, -0.000000000000000000 ) ) ;
#8834=DIRECTION ( 'NONE',  ( 0.000000000000000000, 1.000000000000000000, 0.000000000000000000 ) ) ;
#8835=CIRCLE ( 'NONE', #5454, 1.999999999999998224 ) ;
#8836=AXIS2_PLACEMENT_3D ( 'NONE', #408, #2731, #5961 ) ;
#8841=LINE ( 'NONE', #2968, #2511 ) ;
#8843=DIRECTION ( 'NONE',  ( 0.000000000000000000, 0.000000000000000000, -1.000000000000000000 ) ) ;
#8844=ADVANCED_FACE ( 'NONE', ( #3740 ), #4533, .T. ) ;
#8848=DIRECTION ( 'NONE',  ( -1.000000000000000000, 0.000000000000000000, 0.000000000000000000 ) ) ;
#8849=CARTESIAN_POINT ( 'NONE',  ( 0.000000000000000000, -145.1457019118819005, 49.99999999999997868 ) ) ;
#8850=FACE_OUTER_BOUND ( 'NONE', #4332, .T. ) ;
#8856=FACE_OUTER_BOUND ( 'NONE', #6779, .T. ) ;
#8857=EDGE_CURVE ( 'NONE', #1811, #2596, #8612, .T. ) ;
#8858=CARTESIAN_POINT ( 'NONE',  ( -18.34874108452141783, -140.1746510883711778, -24.43989726270230634 ) ) ;
#8860=CIRCLE ( 'NONE', #5637, 2.000000000000001776 ) ;
#8865=EDGE_CURVE ( 'NONE', #2974, #10235, #3904, .T. ) ;
#8869=CARTESIAN_POINT ( 'NONE',  ( 37.22511195853868315, -117.1457019118819005, -23.15769640663939910 ) ) ;
#8871=DIRECTION ( 'NONE',  ( 0.000000000000000000, 1.000000000000000000, 0.000000000000000000 ) ) ;
#8873=EDGE_LOOP ( 'NONE', ( #2074, #2641 ) ) ;
#8874=CARTESIAN_POINT ( 'NONE',  ( -48.00000000000002842, -117.1457019118819005, 23.15769640663938134 ) ) ;
#8876=ORIENTED_EDGE ( 'NONE', *, *, #1007, .F. ) ;
#8877=CARTESIAN_POINT ( 'NONE',  ( 37.22759939293836595, -133.1457019118818721, 25.15769640663938134 ) ) ;
#8878=VERTEX_POINT ( 'NONE', #3952 ) ;
#8884=CARTESIAN_POINT ( 'NONE',  ( 25.15769640663936713, -117.1457019118819005, 47.99999999999997868 ) ) ;
#8885=CARTESIAN_POINT ( 'NONE',  ( 14.70649310359190309, 120.5696653505793705, 20.00000000000000711 ) ) ;
#8886=CARTESIAN_POINT ( 'NONE',  ( -27.15769640663940976, -117.1457019118819005, 27.15769640663938489 ) ) ;
#8888=ADVANCED_FACE ( 'NONE', ( #5535 ), #7864, .T. ) ;
#8890=ORIENTED_EDGE ( 'NONE', *, *, #1019, .T. ) ;
#8892=EDGE_LOOP ( 'NONE', ( #8719, #1749, #8215, #9447, #8810, #145, #1761, #5570, #8488, #3232, #2687, #2491 ) ) ;
#8896=CARTESIAN_POINT ( 'NONE',  ( -23.76520584195948516, -145.1457019118819005, 49.99999999999997868 ) ) ;
#8897=CARTESIAN_POINT ( 'NONE',  ( -27.15769640663939555, -115.1457019118818863, -27.15769640663944173 ) ) ;
#8898=AXIS2_PLACEMENT_3D ( 'NONE', #6551, #1782, #6606 ) ;
#8899=DIRECTION ( 'NONE',  ( 0.000000000000000000, 0.000000000000000000, 1.000000000000000000 ) ) ;
#8901=VERTEX_POINT ( 'NONE', #666 ) ;
#8902=ADVANCED_FACE ( 'NONE', ( #7871 ), #3098, .T. ) ;
#8903=EDGE_CURVE ( 'NONE', #5352, #1218, #5028, .T. ) ;
#8904=ORIENTED_EDGE ( 'NONE', *, *, #9950, .T. ) ;
#8905=AXIS2_PLACEMENT_3D ( 'NONE', #5072, #5280, #7624 ) ;
#8906=ADVANCED_FACE ( 'NONE', ( #7183 ), #3794, .F. ) ;
#8908=VECTOR ( 'NONE', #4313, 1000.000000000000114 ) ;
#8909=ORIENTED_EDGE ( 'NONE', *, *, #103, .T. ) ;
#8915=DIRECTION ( 'NONE',  ( -1.000000000000000000, 0.000000000000000000, -0.000000000000000000 ) ) ;
#8919=EDGE_CURVE ( 'NONE', #9452, #8605, #4140, .T. ) ;
#8920=CIRCLE ( 'NONE', #4174, 3.999999999999996447 ) ;
#8921=ORIENTED_EDGE ( 'NONE', *, *, #3538, .T. ) ;
#8922=ORIENTED_EDGE ( 'NONE', *, *, #7480, .T. ) ;
#8925=DIRECTION ( 'NONE',  ( -0.000000000000000000, 1.000000000000000000, -0.000000000000000000 ) ) ;
#8927=CARTESIAN_POINT ( 'NONE',  ( 17.97972049165455388, 17.84145331825995484, 25.00000000000000000 ) ) ;
#8928=CIRCLE ( 'NONE', #2662, 4.025000000000000355 ) ;
#8933=EDGE_LOOP ( 'NONE', ( #246, #3773 ) ) ;
#8934=DIRECTION ( 'NONE',  ( -0.000000000000000000, 1.000000000000000000, 0.000000000000000000 ) ) ;
#8937=EDGE_CURVE ( 'NONE', #732, #4565, #8201, .T. ) ;
#8941=FACE_OUTER_BOUND ( 'NONE', #5780, .T. ) ;
#8943=AXIS2_PLACEMENT_3D ( 'NONE', #8742, #530, #2333 ) ;
#8944=ORIENTED_EDGE ( 'NONE', *, *, #4037, .F. ) ;
#8950=CYLINDRICAL_SURFACE ( 'NONE', #5735, 2.000000000000001776 ) ;
#8952=EDGE_CURVE ( 'NONE', #7357, #9778, #3250, .T. ) ;
#8953=DIRECTION ( 'NONE',  ( 0.000000000000000000, 0.000000000000000000, -1.000000000000000000 ) ) ;
#8954=DIRECTION ( 'NONE',  ( 0.000000000000000000, 0.000000000000000000, -1.000000000000000000 ) ) ;
#8955=VECTOR ( 'NONE', #2448, 1000.000000000000000 ) ;
#8959=ORIENTED_EDGE ( 'NONE', *, *, #4829, .F. ) ;
#8960=AXIS2_PLACEMENT_3D ( 'NONE', #7360, #9811, #162 ) ;
#8963=ORIENTED_EDGE ( 'NONE', *, *, #9237, .F. ) ;
#8967=EDGE_CURVE ( 'NONE', #7130, #6316, #7355, .T. ) ;
#8968=EDGE_CURVE ( 'NONE', #8878, #7051, #6427, .T. ) ;
#8972=VERTEX_POINT ( 'NONE', #8019 ) ;
#8974=LINE ( 'NONE', #9130, #129 ) ;
#8976=CARTESIAN_POINT ( 'NONE',  ( 59.99999999999997868, -135.1457019118818721, 40.00000000000000000 ) ) ;
#8977=CYLINDRICAL_SURFACE ( 'NONE', #6124, 2.000000000000001776 ) ;
#8982=DIRECTION ( 'NONE',  ( -0.000000000000000000, -0.000000000000000000, -1.000000000000000000 ) ) ;
#8983=VERTEX_POINT ( 'NONE', #862 ) ;
#8984=CYLINDRICAL_SURFACE ( 'NONE', #864, 3.999999999999989786 ) ;
#8985=ORIENTED_EDGE ( 'NONE', *, *, #9751, .T. ) ;
#8986=CARTESIAN_POINT ( 'NONE',  ( -25.28853996896956957, -134.8487302617674857, 49.99999999999998579 ) ) ;
#8987=ORIENTED_EDGE ( 'NONE', *, *, #9438, .F. ) ;
#8988=SPHERICAL_SURFACE ( 'NONE', #9614, 2.000000000000000000 ) ;
#8989=AXIS2_PLACEMENT_3D ( 'NONE', #9485, #5496, #7102 ) ;
#8990=DIRECTION ( 'NONE',  ( 0.000000000000000000, 0.7071067811864494290, 0.7071067811866454944 ) ) ;
#8991=CARTESIAN_POINT ( 'NONE',  ( 4.856471286862175774, 152.5696653505793279, 30.00000000000000355 ) ) ;
#8997=AXIS2_PLACEMENT_3D ( 'NONE', #7599, #1969, #1918 ) ;
#8998=ORIENTED_EDGE ( 'NONE', *, *, #9679, .T. ) ;
#9000=CARTESIAN_POINT ( 'NONE',  ( 37.59878849545336976, 32.08684478514406635, -12.49999999999999289 ) ) ;
#9002=LINE ( 'NONE', #8148, #235 ) ;
#9004=CIRCLE ( 'NONE', #4101, 4.000000000000000000 ) ;
#9005=DIRECTION ( 'NONE',  ( -0.000000000000000000, 0.000000000000000000, 1.000000000000000000 ) ) ;
#9006=VECTOR ( 'NONE', #9618, 1000.000000000000227 ) ;
#9014=CARTESIAN_POINT ( 'NONE',  ( 23.15769640663936713, -117.1457019118819005, 47.99999999999997868 ) ) ;
#9017=ORIENTED_EDGE ( 'NONE', *, *, #371, .F. ) ;
#9018=DIRECTION ( 'NONE',  ( 0.000000000000000000, 0.000000000000000000, -1.000000000000000000 ) ) ;
#9019=AXIS2_PLACEMENT_3D ( 'NONE', #4470, #1287, #10037 ) ;
#9020=ORIENTED_EDGE ( 'NONE', *, *, #1787, .F. ) ;
#9024=ORIENTED_EDGE ( 'NONE', *, *, #1456, .T. ) ;
#9026=FACE_BOUND ( 'NONE', #8933, .T. ) ;
#9028=CARTESIAN_POINT ( 'NONE',  ( -50.00000000000002132, -117.1457019118819005, 23.15769640663938134 ) ) ;
#9029=CARTESIAN_POINT ( 'NONE',  ( -40.00000000000002842, -135.1457019118818721, 44.02499999999997726 ) ) ;
#9033=DIRECTION ( 'NONE',  ( 0.000000000000000000, 0.000000000000000000, -1.000000000000000000 ) ) ;
#9035=EDGE_CURVE ( 'NONE', #109, #1323, #8022, .T. ) ;
#9036=ORIENTED_EDGE ( 'NONE', *, *, #6169, .T. ) ;
#9039=ADVANCED_FACE ( 'NONE', ( #818 ), #2455, .F. ) ;
#9041=ORIENTED_EDGE ( 'NONE', *, *, #2443, .T. ) ;
#9042=AXIS2_PLACEMENT_3D ( 'NONE', #8296, #6010, #1089 ) ;
#9043=CARTESIAN_POINT ( 'NONE',  ( 25.15769640663938134, -135.1457019118818721, -27.15769640663941331 ) ) ;
#9046=DIRECTION ( 'NONE',  ( -1.000000000000000000, -0.000000000000000000, 0.000000000000000000 ) ) ;
#9047=ORIENTED_EDGE ( 'NONE', *, *, #4646, .T. ) ;
#9056=CARTESIAN_POINT ( 'NONE',  ( 39.99999999999998579, -145.1457019118819005, -40.00000000000002132 ) ) ;
#9060=ORIENTED_EDGE ( 'NONE', *, *, #8857, .F. ) ;
#9061=LINE ( 'NONE', #9714, #1320 ) ;
#9062=AXIS2_PLACEMENT_3D ( 'NONE', #2634, #5750, #8248 ) ;
#9063=DIRECTION ( 'NONE',  ( 0.000000000000000000, 0.000000000000000000, 1.000000000000000000 ) ) ;
#9064=EDGE_CURVE ( 'NONE', #7484, #3453, #2951, .T. ) ;
#9070=DIRECTION ( 'NONE',  ( 1.000000000000000000, 0.000000000000000000, -0.000000000000000000 ) ) ;
#9071=AXIS2_PLACEMENT_3D ( 'NONE', #2565, #4211, #7337 ) ;
#9074=LINE ( 'NONE', #8282, #3005 ) ;
#9075=DIRECTION ( 'NONE',  ( -1.000000000000000000, 0.000000000000000000, 0.000000000000000000 ) ) ;
#9077=CARTESIAN_POINT ( 'NONE',  ( 59.99999999999999289, -135.1457019118818721, -40.00000000000000000 ) ) ;
#9078=CARTESIAN_POINT ( 'NONE',  ( 39.99999999999997158, -145.1457019118819005, 39.99999999999997868 ) ) ;
#9081=ADVANCED_FACE ( 'NONE', ( #6593 ), #9840, .F. ) ;
#9082=CARTESIAN_POINT ( 'NONE',  ( 18.34874108452142494, -140.1746510883711778, -50.00000000000002132 ) ) ;
#9084=DIRECTION ( 'NONE',  ( 0.000000000000000000, -0.000000000000000000, 1.000000000000000000 ) ) ;
#9085=AXIS2_PLACEMENT_3D ( 'NONE', #5651, #685, #3922 ) ;
#9087=CARTESIAN_POINT ( 'NONE',  ( -23.15769640663940976, -133.1457019118818721, 49.99999999999997868 ) ) ;
#9090=ORIENTED_EDGE ( 'NONE', *, *, #8806, .F. ) ;
#9091=VECTOR ( 'NONE', #7763, 1000.000000000000000 ) ;
#9093=DIRECTION ( 'NONE',  ( 0.000000000000000000, 0.000000000000000000, 1.000000000000000000 ) ) ;
#9099=AXIS2_PLACEMENT_3D ( 'NONE', #6147, #5193, #8430 ) ;
#9100=CARTESIAN_POINT ( 'NONE',  ( -18.34874108452141783, -140.1746510883711778, 24.43989726270226370 ) ) ;
#9101=ORIENTED_EDGE ( 'NONE', *, *, #7195, .F. ) ;
#9102=AXIS2_PLACEMENT_3D ( 'NONE', #6317, #9666, #9617 ) ;
#9105=CARTESIAN_POINT ( 'NONE',  ( -16.29350689640809691, -115.1457019118818863, -23.72119897386845722 ) ) ;
#9106=CARTESIAN_POINT ( 'NONE',  ( -23.15769640663940265, -117.1457019118819005, -3.234176690190487260E-15 ) ) ;
#9110=AXIS2_PLACEMENT_3D ( 'NONE', #3878, #10343, #3928 ) ;
#9112=CYLINDRICAL_SURFACE ( 'NONE', #9392, 2.000000000000001776 ) ;
#9118=DIRECTION ( 'NONE',  ( 0.000000000000000000, 0.000000000000000000, 1.000000000000000000 ) ) ;
#9119=DIRECTION ( 'NONE',  ( 1.000000000000000000, 0.000000000000000000, 0.000000000000000000 ) ) ;
#9123=ORIENTED_EDGE ( 'NONE', *, *, #2111, .T. ) ;
#9130=CARTESIAN_POINT ( 'NONE',  ( -23.15769640663940976, -115.1457019118818863, -1.617088345095243827E-14 ) ) ;
#9132=LINE ( 'NONE', #8177, #6871 ) ;
#9133=DIRECTION ( 'NONE',  ( 1.000000000000000000, 0.000000000000000000, 0.000000000000000000 ) ) ;
#9134=VECTOR ( 'NONE', #8522, 1000.000000000000000 ) ;
#9136=CARTESIAN_POINT ( 'NONE',  ( 37.23187270759618883, -133.8059336968422883, -25.26512318821856340 ) ) ;
#9139=ORIENTED_EDGE ( 'NONE', *, *, #1306, .F. ) ;
#9142=ORIENTED_EDGE ( 'NONE', *, *, #9653, .T. ) ;
#9143=CARTESIAN_POINT ( 'NONE',  ( 39.99999999999998579, -145.1457019118819005, -40.00000000000002132 ) ) ;
#9149=ORIENTED_EDGE ( 'NONE', *, *, #10385, .T. ) ;
#9151=EDGE_CURVE ( 'NONE', #9794, #7113, #1332, .T. ) ;
#9153=AXIS2_PLACEMENT_3D ( 'NONE', #8886, #2525, #8138 ) ;
#9154=ORIENTED_EDGE ( 'NONE', *, *, #8378, .T. ) ;
#9155=DIRECTION ( 'NONE',  ( 0.000000000000000000, 0.000000000000000000, 1.000000000000000000 ) ) ;
#9156=CARTESIAN_POINT ( 'NONE',  ( -2.293506896408097795, 37.08684478514406635, 30.00000000000000355 ) ) ;
#9157=DIRECTION ( 'NONE',  ( 0.000000000000000000, -1.000000000000000000, 0.000000000000000000 ) ) ;
#9159=CARTESIAN_POINT ( 'NONE',  ( 39.99999999999997158, -135.1457019118818721, 39.99999999999997868 ) ) ;
#9160=DIRECTION ( 'NONE',  ( -1.000000000000000000, -0.000000000000000000, -8.379529552680125332E-16 ) ) ;
#9164=ORIENTED_EDGE ( 'NONE', *, *, #4724, .F. ) ;
#9165=EDGE_CURVE ( 'NONE', #3261, #5755, #6501, .T. ) ;
#9168=DIRECTION ( 'NONE',  ( -1.000000000000000000, 0.000000000000000000, 0.000000000000000000 ) ) ;
#9169=PLANE ( 'NONE',  #3590 ) ;
#9171=( GEOMETRIC_REPRESENTATION_CONTEXT ( 3 ) GLOBAL_UNCERTAINTY_ASSIGNED_CONTEXT ( ( #75 ) ) GLOBAL_UNIT_ASSIGNED_CONTEXT ( ( #6894, #10132, #9981 ) ) REPRESENTATION_CONTEXT ( 'NONE', 'WORKASPACE' ) );
#9175=FACE_OUTER_BOUND ( 'NONE', #696, .T. ) ;
#9177=CYLINDRICAL_SURFACE ( 'NONE', #4889, 4.000000000000000000 ) ;
#9178=CIRCLE ( 'NONE', #6634, 2.000000000000001776 ) ;
#9179=AXIS2_PLACEMENT_3D ( 'NONE', #6280, #9635, #5484 ) ;
#9185=FACE_OUTER_BOUND ( 'NONE', #1231, .T. ) ;
#9186=CARTESIAN_POINT ( 'NONE',  ( -16.29350689640809691, -140.1746510883711778, 0.000000000000000000 ) ) ;
#9187=VECTOR ( 'NONE', #7647, 1000.000000000000000 ) ;
#9190=EDGE_CURVE ( 'NONE', #8878, #7930, #6203, .T. ) ;
#9193=CARTESIAN_POINT ( 'NONE',  ( 4.856471286862175774, 147.5696653505793279, -30.00000000000000355 ) ) ;
#9194=ORIENTED_EDGE ( 'NONE', *, *, #2895, .T. ) ;
#9195=VECTOR ( 'NONE', #6256, 1000.000000000000000 ) ;
#9196=CYLINDRICAL_SURFACE ( 'NONE', #7104, 2.000000000000001776 ) ;
#9204=AXIS2_PLACEMENT_3D ( 'NONE', #3072, #4029, #2228 ) ;
#9208=CARTESIAN_POINT ( 'NONE',  ( -38.19229777560033057, 152.5696653505793279, 12.50000000000000000 ) ) ;
#9211=EDGE_LOOP ( 'NONE', ( #1227, #6988, #4897, #3442 ) ) ;
#9212=SPHERICAL_SURFACE ( 'NONE', #282, 2.000000000000000000 ) ;
#9213=CARTESIAN_POINT ( 'NONE',  ( 99.80027788547049283, -145.1457019118819005, -24.99999999999998934 ) ) ;
#9215=PLANE ( 'NONE',  #1 ) ;
#9216=CARTESIAN_POINT ( 'NONE',  ( 33.55285093437175448, 29.14909237014566301, -12.50000000000000000 ) ) ;
#9218=DIRECTION ( 'NONE',  ( 0.000000000000000000, 0.000000000000000000, 1.000000000000000000 ) ) ;
#9225=LINE ( 'NONE', #8536, #4118 ) ;
#9226=DIRECTION ( 'NONE',  ( 0.000000000000000000, -1.000000000000000000, 0.000000000000000000 ) ) ;
#9227=ORIENTED_EDGE ( 'NONE', *, *, #964, .F. ) ;
#9231=ADVANCED_FACE ( 'NONE', ( #3931 ), #2113, .T. ) ;
#9234=ORIENTED_EDGE ( 'NONE', *, *, #6086, .T. ) ;
#9235=LINE ( 'NONE', #10034, #5547 ) ;
#9237=EDGE_CURVE ( 'NONE', #6945, #3843, #8001, .T. ) ;
#9239=DIRECTION ( 'NONE',  ( 0.000000000000000000, 0.000000000000000000, -1.000000000000000000 ) ) ;
#9240=AXIS2_PLACEMENT_3D ( 'NONE', #6640, #7600, #3303 ) ;
#9243=ADVANCED_FACE ( 'NONE', ( #8850 ), #3074, .T. ) ;
#9245=DIRECTION ( 'NONE',  ( 0.000000000000000000, 0.000000000000000000, -1.000000000000000000 ) ) ;
#9246=ORIENTED_EDGE ( 'NONE', *, *, #8968, .T. ) ;
#9247=AXIS2_PLACEMENT_3D ( 'NONE', #3679, #4622, #2766 ) ;
#9249=FACE_OUTER_BOUND ( 'NONE', #1694, .T. ) ;
#9250=CIRCLE ( 'NONE', #10100, 19.24539146688411506 ) ;
#9252=DIRECTION ( 'NONE',  ( -1.000000000000000000, -0.000000000000000000, -0.000000000000000000 ) ) ;
#9255=ORIENTED_EDGE ( 'NONE', *, *, #8736, .F. ) ;
#9256=FACE_OUTER_BOUND ( 'NONE', #9634, .T. ) ;
#9259=EDGE_LOOP ( 'NONE', ( #3310, #6239, #9354, #6778 ) ) ;
#9261=EDGE_CURVE ( 'NONE', #8972, #426, #2286, .T. ) ;
#9262=TOROIDAL_SURFACE ( 'NONE', #10455, 4.000000000000000000, 2.000000000000000000 ) ;
#9265=DIRECTION ( 'NONE',  ( 0.000000000000000000, 0.000000000000000000, -1.000000000000000000 ) ) ;
#9269=DIRECTION ( 'NONE',  ( -1.000000000000000000, 0.000000000000000000, -0.000000000000000000 ) ) ;
#9271=CYLINDRICAL_SURFACE ( 'NONE', #7970, 3.999999999999989786 ) ;
#9272=AXIS2_PLACEMENT_3D ( 'NONE', #9726, #4782, #1608 ) ;
#9274=ORIENTED_EDGE ( 'NONE', *, *, #3776, .T. ) ;
#9275=FACE_OUTER_BOUND ( 'NONE', #207, .T. ) ;
#9280=CIRCLE ( 'NONE', #1823, 3.999999999999989786 ) ;
#9283=CIRCLE ( 'NONE', #5386, 2.000000000000001776 ) ;
#9286=CARTESIAN_POINT ( 'NONE',  ( -40.00000000000001421, -135.1457019118818721, -44.02500000000001990 ) ) ;
#9287=VECTOR ( 'NONE', #4506, 1000.000000000000000 ) ;
#9290=ADVANCED_FACE ( 'NONE', ( #7211 ), #5567, .T. ) ;
#9291=DIRECTION ( 'NONE',  ( -0.000000000000000000, 1.000000000000000000, -0.000000000000000000 ) ) ;
#9292=LINE ( 'NONE', #7800, #535 ) ;
#9293=EDGE_CURVE ( 'NONE', #7537, #10220, #928, .T. ) ;
#9295=PLANE ( 'NONE',  #1127 ) ;
#9297=CARTESIAN_POINT ( 'NONE',  ( -40.00000000000001421, -135.1457019118818721, -35.97500000000002274 ) ) ;
#9302=PRODUCT_DEFINITION ( 'UNKNOWN', '', #1431, #7489 ) ;
#9303=VERTEX_POINT ( 'NONE', #3227 ) ;
#9304=EDGE_CURVE ( 'NONE', #1323, #109, #3815, .T. ) ;
#9305=EDGE_CURVE ( 'NONE', #6600, #7930, #4866, .T. ) ;
#9311=CARTESIAN_POINT ( 'NONE',  ( 14.70649310359190309, 80.56966535057935630, 20.00000000000000711 ) ) ;
#9312=ORIENTED_EDGE ( 'NONE', *, *, #414, .T. ) ;
#9317=CARTESIAN_POINT ( 'NONE',  ( -50.00000000000002132, -115.1457019118818863, -23.15769640663945594 ) ) ;
#9320=FACE_OUTER_BOUND ( 'NONE', #7451, .T. ) ;
#9323=DIRECTION ( 'NONE',  ( 0.000000000000000000, 0.000000000000000000, 1.000000000000000000 ) ) ;
#9330=VECTOR ( 'NONE', #2853, 1000.000000000000000 ) ;
#9334=DIRECTION ( 'NONE',  ( 0.000000000000000000, 0.000000000000000000, 1.000000000000000000 ) ) ;
#9335=CARTESIAN_POINT ( 'NONE',  ( 37.22511195853869026, -115.1457019118818863, 23.15769640663938134 ) ) ;
#9340=AXIS2_PLACEMENT_3D ( 'NONE', #599, #7069, #3035 ) ;
#9343=LINE ( 'NONE', #1968, #139 ) ;
#9345=LINE ( 'NONE', #6796, #10439 ) ;
#9347=DIRECTION ( 'NONE',  ( 1.000000000000000000, -1.802741689055041147E-15, 0.000000000000000000 ) ) ;
#9351=( BOUNDED_CURVE ( )  B_SPLINE_CURVE ( 3, ( #3319, #5061, #7346, #7295 ),
 .UNSPECIFIED., .F., .T. ) 
 B_SPLINE_CURVE_WITH_KNOTS ( ( 4, 4 ),
 ( 1.848378549510505620, 3.054692141489262713 ),
 .UNSPECIFIED. ) 
 CURVE ( )  GEOMETRIC_REPRESENTATION_ITEM ( )  RATIONAL_B_SPLINE_CURVE ( ( 1.000000000000000000, 0.8823660295963220435, 0.8823660295963220435, 1.000000000000000000 ) ) 
 REPRESENTATION_ITEM ( '' )  );
#9352=ADVANCED_FACE ( 'NONE', ( #6513 ), #5819, .F. ) ;
#9353=FACE_OUTER_BOUND ( 'NONE', #3646, .T. ) ;
#9354=ORIENTED_EDGE ( 'NONE', *, *, #7267, .F. ) ;
#9357=CARTESIAN_POINT ( 'NONE',  ( -40.00000000000002842, -135.1457019118818721, 35.97499999999998010 ) ) ;
#9359=CARTESIAN_POINT ( 'NONE',  ( -2.293506896408097795, 120.5696653505793705, -24.00000000000000711 ) ) ;
#9360=ORIENTED_EDGE ( 'NONE', *, *, #1696, .T. ) ;
#9361=CARTESIAN_POINT ( 'NONE',  ( 37.22759939293836595, -117.1457019118819005, 25.15769640663938134 ) ) ;
#9363=EDGE_CURVE ( 'NONE', #7873, #1605, #4968, .T. ) ;
#9365=EDGE_CURVE ( 'NONE', #9778, #4565, #595, .T. ) ;
#9368=FACE_OUTER_BOUND ( 'NONE', #8333, .T. ) ;
#9369=ORIENTED_EDGE ( 'NONE', *, *, #3266, .F. ) ;
#9371=DIRECTION ( 'NONE',  ( -1.000000000000000000, -0.000000000000000000, 0.000000000000000000 ) ) ;
#9372=DIRECTION ( 'NONE',  ( -0.000000000000000000, -0.000000000000000000, -1.000000000000000000 ) ) ;
#9375=DIRECTION ( 'NONE',  ( 8.659560562356134638E-17, 0.7071067811864494290, -0.7071067811866454944 ) ) ;
#9376=DIRECTION ( 'NONE',  ( 0.000000000000000000, 0.000000000000000000, -1.000000000000000000 ) ) ;
#9378=DIRECTION ( 'NONE',  ( -0.000000000000000000, 1.000000000000000000, -0.000000000000000000 ) ) ;
#9379=EDGE_CURVE ( 'NONE', #6373, #6699, #8030, .T. ) ;
#9383=CARTESIAN_POINT ( 'NONE',  ( 14.70649310359190309, 120.5696653505793705, 20.00000000000000711 ) ) ;
#9385=CARTESIAN_POINT ( 'NONE',  ( 23.15769640663938134, -117.1457019118819005, -27.15769640663941686 ) ) ;
#9386=CARTESIAN_POINT ( 'NONE',  ( 37.22511195853869026, -115.1457019118818863, -23.15769640663939910 ) ) ;
#9388=AXIS2_PLACEMENT_3D ( 'NONE', #4103, #7335, #1715 ) ;
#9390=ORIENTED_EDGE ( 'NONE', *, *, #6234, .F. ) ;
#9392=AXIS2_PLACEMENT_3D ( 'NONE', #5761, #1002, #896 ) ;
#9393=ORIENTED_EDGE ( 'NONE', *, *, #4215, .T. ) ;
#9396=EDGE_CURVE ( 'NONE', #4437, #5933, #7869, .T. ) ;
#9399=CARTESIAN_POINT ( 'NONE',  ( 38.19229777560031636, 118.3760186273086816, 12.50000000000000000 ) ) ;
#9401=ORIENTED_EDGE ( 'NONE', *, *, #5082, .T. ) ;
#9403=CYLINDRICAL_SURFACE ( 'NONE', #6921, 2.000000000000001776 ) ;
#9404=EDGE_LOOP ( 'NONE', ( #8909, #10083, #5538 ) ) ;
#9407=ADVANCED_FACE ( 'NONE', ( #3493 ), #9112, .F. ) ;
#9411=CARTESIAN_POINT ( 'NONE',  ( 37.22759939293836595, -117.1457019118819005, 25.15769640663938134 ) ) ;
#9412=ORIENTED_EDGE ( 'NONE', *, *, #332, .F. ) ;
#9413=DIRECTION ( 'NONE',  ( 0.000000000000000000, 0.000000000000000000, -1.000000000000000000 ) ) ;
#9417=ORIENTED_EDGE ( 'NONE', *, *, #5270, .F. ) ;
#9423=EDGE_CURVE ( 'NONE', #3840, #8901, #8715, .T. ) ;
#9428=CARTESIAN_POINT ( 'NONE',  ( -23.76520584195948516, -145.1457019118819005, -97.78965767959371647 ) ) ;
#9430=CARTESIAN_POINT ( 'NONE',  ( -48.00000000000002132, -133.1457019118818721, -23.15769640663945594 ) ) ;
#9431=CIRCLE ( 'NONE', #6033, 4.999999999999995559 ) ;
#9434=ORIENTED_EDGE ( 'NONE', *, *, #964, .T. ) ;
#9435=CIRCLE ( 'NONE', #2656, 3.999999999999989786 ) ;
#9438=EDGE_CURVE ( 'NONE', #8738, #2339, #3644, .T. ) ;
#9439=FACE_OUTER_BOUND ( 'NONE', #3272, .T. ) ;
#9442=EDGE_CURVE ( 'NONE', #2474, #8605, #57, .T. ) ;
#9443=CARTESIAN_POINT ( 'NONE',  ( -50.00000000000002842, -134.6884760388430777, 24.98775663295401372 ) ) ;
#9444=CARTESIAN_POINT ( 'NONE',  ( -2.293506896408097795, 80.56966535057935630, -16.00000000000000711 ) ) ;
#9447=ORIENTED_EDGE ( 'NONE', *, *, #287, .T. ) ;
#9448=VERTEX_POINT ( 'NONE', #4075 ) ;
#9452=VERTEX_POINT ( 'NONE', #215 ) ;
#9454=CARTESIAN_POINT ( 'NONE',  ( 23.39899473324886614, -133.3869996355172987, 49.99999999999998579 ) ) ;
#9455=DIRECTION ( 'NONE',  ( -1.000000000000000000, -0.000000000000000000, 0.000000000000000000 ) ) ;
#9457=CARTESIAN_POINT ( 'NONE',  ( 23.15769640663940265, -133.1457019118818721, -50.00000000000002132 ) ) ;
#9459=VERTEX_POINT ( 'NONE', #2537 ) ;
#9460=CARTESIAN_POINT ( 'NONE',  ( 77.30044127146540234, 73.68369600860394542, -24.99999999999998934 ) ) ;
#9463=LINE ( 'NONE', #8500, #5026 ) ;
#9464=DIRECTION ( 'NONE',  ( 0.6585271261848804070, -0.7525569905852198538, 0.000000000000000000 ) ) ;
#9466=CARTESIAN_POINT ( 'NONE',  ( 23.64292728780886321, -133.6309146189979060, -50.00000000000002842 ) ) ;
#9468=ORIENTED_EDGE ( 'NONE', *, *, #373, .F. ) ;
#9470=ORIENTED_EDGE ( 'NONE', *, *, #2200, .F. ) ;
#9476=ORIENTED_EDGE ( 'NONE', *, *, #3024, .T. ) ;
#9477=VERTEX_POINT ( 'NONE', #5870 ) ;
#9478=CARTESIAN_POINT ( 'NONE',  ( -16.29350689640809691, -186.9457019118818835, -30.31717237747080773 ) ) ;
#9479=CARTESIAN_POINT ( 'NONE',  ( 37.22759939293836595, -135.1457019118818721, 25.15769640663938134 ) ) ;
#9483=ADVANCED_FACE ( 'NONE', ( #5975 ), #6993, .T. ) ;
#9484=CARTESIAN_POINT ( 'NONE',  ( -23.15769640663940976, -133.1457019118818721, 47.99999999999997868 ) ) ;
#9485=CARTESIAN_POINT ( 'NONE',  ( 37.22511195853869026, -145.1457019118819005, 30.00000000000000355 ) ) ;
#9487=EDGE_CURVE ( 'NONE', #9303, #10082, #10354, .T. ) ;
#9490=CARTESIAN_POINT ( 'NONE',  ( -25.15769640663937423, -135.1457019118818721, -48.00000000000002132 ) ) ;
#9491=VERTEX_POINT ( 'NONE', #4398 ) ;
#9492=DIRECTION ( 'NONE',  ( 0.07334937666141724821, -0.9973063064792989652, -0.000000000000000000 ) ) ;
#9497=CARTESIAN_POINT ( 'NONE',  ( 38.19229777560031636, -43.28483205141633761, 12.50000000000000000 ) ) ;
#9498=DIRECTION ( 'NONE',  ( 0.000000000000000000, 1.000000000000000000, 0.000000000000000000 ) ) ;
#9499=EDGE_LOOP ( 'NONE', ( #1202, #6533, #2349, #2969 ) ) ;
#9500=ORIENTED_EDGE ( 'NONE', *, *, #7208, .T. ) ;
#9505=ORIENTED_EDGE ( 'NONE', *, *, #8261, .F. ) ;
#9509=VECTOR ( 'NONE', #201, 1000.000000000000000 ) ;
#9510=DIRECTION ( 'NONE',  ( 0.7525569905852205199, 0.6585271261848794078, 0.000000000000000000 ) ) ;
#9515=AXIS2_PLACEMENT_3D ( 'NONE', #7761, #6801, #9245 ) ;
#9518=AXIS2_PLACEMENT_3D ( 'NONE', #969, #4306, #7541 ) ;
#9521=EDGE_CURVE ( 'NONE', #5490, #3561, #1204, .T. ) ;
#9523=AXIS2_PLACEMENT_3D ( 'NONE', #7962, #6318, #8701 ) ;
#9527=CYLINDRICAL_SURFACE ( 'NONE', #8160, 2.000000000000001776 ) ;
#9531=CARTESIAN_POINT ( 'NONE',  ( -27.15769640663940976, -117.1457019118819005, 25.15769640663938134 ) ) ;
#9533=ORIENTED_EDGE ( 'NONE', *, *, #3837, .T. ) ;
#9534=VERTEX_POINT ( 'NONE', #6830 ) ;
#9535=CARTESIAN_POINT ( 'NONE',  ( 25.15769640663938134, -117.1457019118819005, -27.15769640663941331 ) ) ;
#9536=CARTESIAN_POINT ( 'NONE',  ( 25.15769640663936713, -115.1457019118818863, 47.99999999999997868 ) ) ;
#9538=DIRECTION ( 'NONE',  ( -1.000000000000000000, 0.000000000000000000, 0.000000000000000000 ) ) ;
#9542=DIRECTION ( 'NONE',  ( -1.000000000000000000, -1.734723475976801918E-16, 1.734723475976813997E-16 ) ) ;
#9543=VECTOR ( 'NONE', #10041, 1000.000000000000000 ) ;
#9552=CARTESIAN_POINT ( 'NONE',  ( -18.34874108452141783, -140.1746510883711778, -97.78965767959371647 ) ) ;
#9553=EDGE_CURVE ( 'NONE', #1218, #6270, #1211, .T. ) ;
#9554=CARTESIAN_POINT ( 'NONE',  ( 14.70649310359190309, 120.5696653505793705, -20.00000000000000711 ) ) ;
#9555=DIRECTION ( 'NONE',  ( -6.982941293900105430E-16, 0.000000000000000000, 1.000000000000000000 ) ) ;
#9556=VERTEX_POINT ( 'NONE', #2054 ) ;
#9560=ORIENTED_EDGE ( 'NONE', *, *, #8300, .T. ) ;
#9561=ORIENTED_EDGE ( 'NONE', *, *, #7327, .F. ) ;
#9562=CARTESIAN_POINT ( 'NONE',  ( 37.22511195853866894, 17.84145331825995484, 30.00000000000000355 ) ) ;
#9564=AXIS2_PLACEMENT_3D ( 'NONE', #9799, #5854, #9093 ) ;
#9567=ADVANCED_FACE ( 'NONE', ( #6028 ), #9271, .F. ) ;
#9568=EDGE_CURVE ( 'NONE', #1563, #6846, #4448, .T. ) ;
#9570=DIRECTION ( 'NONE',  ( 0.000000000000000000, 0.000000000000000000, 1.000000000000000000 ) ) ;
#9572=CYLINDRICAL_SURFACE ( 'NONE', #10360, 19.24539146688411506 ) ;
#9574=ORIENTED_EDGE ( 'NONE', *, *, #3459, .T. ) ;
#9577=VECTOR ( 'NONE', #7117, 1000.000000000000000 ) ;
#9579=CARTESIAN_POINT ( 'NONE',  ( 17.97972049165455388, 42.08684478514406635, 25.00000000000000000 ) ) ;
#9580=CARTESIAN_POINT ( 'NONE',  ( 37.22511195853866894, 17.84145331825995839, 30.00000000000000355 ) ) ;
#9581=FACE_OUTER_BOUND ( 'NONE', #4499, .T. ) ;
#9582=VERTEX_POINT ( 'NONE', #1533 ) ;
#9583=DIRECTION ( 'NONE',  ( 1.000000000000000000, -0.000000000000000000, 0.000000000000000000 ) ) ;
#9586=DIRECTION ( 'NONE',  ( -0.000000000000000000, 1.000000000000000000, -0.000000000000000000 ) ) ;
#9587=EDGE_LOOP ( 'NONE', ( #6500, #5290, #6769, #2977 ) ) ;
#9588=AXIS2_PLACEMENT_3D ( 'NONE', #7135, #6277, #3850 ) ;
#9592=CARTESIAN_POINT ( 'NONE',  ( 14.70649310359190309, 80.56966535057935630, 20.00000000000000711 ) ) ;
#9597=PRODUCT_DEFINITION_SHAPE ( 'NONE', 'NONE',  #9302 ) ;
#9599=ADVANCED_FACE ( 'NONE', ( #3813 ), #3165, .T. ) ;
#9600=EDGE_LOOP ( 'NONE', ( #2748, #6105 ) ) ;
#9608=FACE_OUTER_BOUND ( 'NONE', #2799, .T. ) ;
#9609=LINE ( 'NONE', #8849, #4659 ) ;
#9614=AXIS2_PLACEMENT_3D ( 'NONE', #1780, #9850, #9733 ) ;
#9616=VERTEX_POINT ( 'NONE', #2216 ) ;
#9617=DIRECTION ( 'NONE',  ( 0.000000000000000000, -0.000000000000000000, -1.000000000000000000 ) ) ;
#9618=DIRECTION ( 'NONE',  ( -0.07334937666141724821, 0.9973063064792989652, 0.000000000000000000 ) ) ;
#9620=CARTESIAN_POINT ( 'NONE',  ( -25.93998375192765948, -135.0799149511624364, -50.00000000000002842 ) ) ;
#9622=CIRCLE ( 'NONE', #3345, 3.999999999999996447 ) ;
#9627=ADVANCED_FACE ( 'NONE', ( #7200 ), #4749, .T. ) ;
#9628=ADVANCED_FACE ( 'NONE', ( #578, #8035, #6348 ), #8734, .F. ) ;
#9632=CARTESIAN_POINT ( 'NONE',  ( 39.99999999999997158, -135.1707019118818778, 39.99999999999997868 ) ) ;
#9634=EDGE_LOOP ( 'NONE', ( #3714, #550, #3640, #4805 ) ) ;
#9635=DIRECTION ( 'NONE',  ( 0.000000000000000000, 1.000000000000000000, 0.000000000000000000 ) ) ;
#9639=EDGE_CURVE ( 'NONE', #2017, #2815, #9674, .T. ) ;
#9642=DIRECTION ( 'NONE',  ( -0.000000000000000000, -0.000000000000000000, 1.000000000000000000 ) ) ;
#9643=ORIENTED_EDGE ( 'NONE', *, *, #1177, .T. ) ;
#9647=DIRECTION ( 'NONE',  ( 1.000000000000000000, 0.000000000000000000, 0.000000000000000000 ) ) ;
#9649=DIRECTION ( 'NONE',  ( 0.000000000000000000, 0.000000000000000000, 1.000000000000000000 ) ) ;
#9650=DIRECTION ( 'NONE',  ( 1.000000000000000000, 0.000000000000000000, 0.000000000000000000 ) ) ;
#9653=EDGE_CURVE ( 'NONE', #8659, #6555, #10179, .T. ) ;
#9654=DIRECTION ( 'NONE',  ( -0.000000000000000000, 1.000000000000000000, -0.000000000000000000 ) ) ;
#9656=DIRECTION ( 'NONE',  ( 0.000000000000000000, 0.000000000000000000, 1.000000000000000000 ) ) ;
#9658=AXIS2_PLACEMENT_3D ( 'NONE', #6827, #5336, #6937 ) ;
#9660=EDGE_CURVE ( 'NONE', #4536, #1149, #5430, .T. ) ;
#9661=CARTESIAN_POINT ( 'NONE',  ( 39.99999999999998579, -135.1457019118818721, -40.00000000000002132 ) ) ;
#9663=ORIENTED_EDGE ( 'NONE', *, *, #5425, .F. ) ;
#9664=ORIENTED_EDGE ( 'NONE', *, *, #7497, .F. ) ;
#9666=DIRECTION ( 'NONE',  ( 0.000000000000000000, -1.000000000000000000, 0.000000000000000000 ) ) ;
#9667=CARTESIAN_POINT ( 'NONE',  ( 26.27514435518734004, -135.1457019118818437, 49.99999999999997158 ) ) ;
#9668=CARTESIAN_POINT ( 'NONE',  ( -26.27514435518734004, -135.1457019118818437, -50.00000000000001421 ) ) ;
#9670=CARTESIAN_POINT ( 'NONE',  ( -40.00000000000001421, -135.1457019118818721, -40.00000000000002132 ) ) ;
#9673=ORIENTED_EDGE ( 'NONE', *, *, #4504, .T. ) ;
#9674=CIRCLE ( 'NONE', #7294, 7.525240063345735031 ) ;
#9679=EDGE_CURVE ( 'NONE', #5755, #5017, #7945, .T. ) ;
#9681=VECTOR ( 'NONE', #4570, 1000.000000000000000 ) ;
#9682=LINE ( 'NONE', #6649, #4084 ) ;
#9689=CARTESIAN_POINT ( 'NONE',  ( -27.15769640663941331, -133.1457019118818721, 47.99999999999997868 ) ) ;
#9690=ADVANCED_FACE ( 'NONE', ( #7890, #7835, #3016 ), #631, .F. ) ;
#9692=CARTESIAN_POINT ( 'NONE',  ( 49.99999999999997158, -145.1457019118819005, 39.99999999999997868 ) ) ;
#9694=DIRECTION ( 'NONE',  ( 0.000000000000000000, 0.000000000000000000, 1.000000000000000000 ) ) ;
#9696=AXIS2_PLACEMENT_3D ( 'NONE', #1250, #6173, #1939 ) ;
#9706=DIRECTION ( 'NONE',  ( -0.000000000000000000, -0.000000000000000000, -1.000000000000000000 ) ) ;
#9707=DIRECTION ( 'NONE',  ( 1.000000000000000000, 0.000000000000000000, 0.000000000000000000 ) ) ;
#9709=ORIENTED_EDGE ( 'NONE', *, *, #6760, .F. ) ;
#9711=ORIENTED_EDGE ( 'NONE', *, *, #7068, .T. ) ;
#9713=EDGE_LOOP ( 'NONE', ( #9574, #3506, #2704, #1432 ) ) ;
#9714=CARTESIAN_POINT ( 'NONE',  ( -50.00000000000002132, -145.1457019118819005, -6.938893903907231533E-15 ) ) ;
#9715=DIRECTION ( 'NONE',  ( 0.000000000000000000, 0.000000000000000000, -1.000000000000000000 ) ) ;
#9723=CIRCLE ( 'NONE', #2276, 5.000000000000002665 ) ;
#9725=ORIENTED_EDGE ( 'NONE', *, *, #373, .T. ) ;
#9726=CARTESIAN_POINT ( 'NONE',  ( -48.00000000000002132, -133.1457019118818721, 23.15769640663938134 ) ) ;
#9728=CARTESIAN_POINT ( 'NONE',  ( -2.293506896408097795, 80.56966535057935630, 16.00000000000000711 ) ) ;
#9730=CARTESIAN_POINT ( 'NONE',  ( 37.60403889007154987, -135.1346877209587376, -26.91386751108004560 ) ) ;
#9731=AXIS2_PLACEMENT_3D ( 'NONE', #3848, #4580, #2310 ) ;
#9733=DIRECTION ( 'NONE',  ( 0.000000000000000000, 0.000000000000000000, -1.000000000000000000 ) ) ;
#9740=VERTEX_POINT ( 'NONE', #3322 ) ;
#9741=DIRECTION ( 'NONE',  ( -0.000000000000000000, -0.000000000000000000, -1.000000000000000000 ) ) ;
#9750=LINE ( 'NONE', #5702, #636 ) ;
#9751=EDGE_CURVE ( 'NONE', #3286, #3513, #8089, .T. ) ;
#9752=ADVANCED_FACE ( 'NONE', ( #830 ), #5763, .F. ) ;
#9753=ORIENTED_EDGE ( 'NONE', *, *, #9751, .F. ) ;
#9757=LINE ( 'NONE', #7260, #4053 ) ;
#9761=DIRECTION ( 'NONE',  ( 0.000000000000000000, 0.000000000000000000, 1.000000000000000000 ) ) ;
#9763=ORIENTED_EDGE ( 'NONE', *, *, #5847, .T. ) ;
#9764=ORIENTED_EDGE ( 'NONE', *, *, #8919, .F. ) ;
#9765=AXIS2_PLACEMENT_3D ( 'NONE', #5231, #7725, #6823 ) ;
#9766=ADVANCED_FACE ( 'NONE', ( #4066 ), #7352, .F. ) ;
#9769=EDGE_CURVE ( 'NONE', #6079, #1518, #2556, .T. ) ;
#9772=FACE_OUTER_BOUND ( 'NONE', #7850, .T. ) ;
#9777=CIRCLE ( 'NONE', #1093, 2.000000000000001776 ) ;
#9778=VERTEX_POINT ( 'NONE', #4851 ) ;
#9779=AXIS2_PLACEMENT_3D ( 'NONE', #876, #8192, #4848 ) ;
#9780=CARTESIAN_POINT ( 'NONE',  ( 37.22511195853866894, 17.84145331825995839, 25.00000000000000000 ) ) ;
#9781=VECTOR ( 'NONE', #3971, 1000.000000000000000 ) ;
#9783=VERTEX_POINT ( 'NONE', #2470 ) ;
#9788=EDGE_CURVE ( 'NONE', #5030, #3054, #2635, .T. ) ;
#9790=ORIENTED_EDGE ( 'NONE', *, *, #10101, .F. ) ;
#9791=LINE ( 'NONE', #2405, #6815 ) ;
#9793=DIRECTION ( 'NONE',  ( 6.982941293900105430E-16, -0.000000000000000000, -1.000000000000000000 ) ) ;
#9794=VERTEX_POINT ( 'NONE', #7297 ) ;
#9796=VECTOR ( 'NONE', #2024, 1000.000000000000000 ) ;
#9798=DIRECTION ( 'NONE',  ( 0.000000000000000000, 0.000000000000000000, 1.000000000000000000 ) ) ;
#9799=CARTESIAN_POINT ( 'NONE',  ( -40.00000000000001421, -135.1457019118818721, -40.00000000000002132 ) ) ;
#9800=DIRECTION ( 'NONE',  ( 0.000000000000000000, -1.000000000000000000, 0.000000000000000000 ) ) ;
#9803=ADVANCED_FACE ( 'NONE', ( #1835 ), #4914, .T. ) ;
#9804=CIRCLE ( 'NONE', #1497, 2.000000000000001776 ) ;
#9805=ORIENTED_EDGE ( 'NONE', *, *, #5317, .T. ) ;
#9808=VERTEX_POINT ( 'NONE', #6711 ) ;
#9811=DIRECTION ( 'NONE',  ( 0.000000000000000000, -1.000000000000000000, 0.000000000000000000 ) ) ;
#9813=CARTESIAN_POINT ( 'NONE',  ( -2.293506896408097795, 37.08684478514406635, 25.00000000000000000 ) ) ;
#9819=ORIENTED_EDGE ( 'NONE', *, *, #1007, .T. ) ;
#9821=VECTOR ( 'NONE', #839, 1000.000000000000000 ) ;
#9828=ADVANCED_FACE ( 'NONE', ( #8941 ), #8249, .T. ) ;
#9829=EDGE_CURVE ( 'NONE', #2596, #1304, #3230, .T. ) ;
#9832=ORIENTED_EDGE ( 'NONE', *, *, #2964, .F. ) ;
#9839=DIRECTION ( 'NONE',  ( -1.000000000000000000, 0.000000000000000000, 0.000000000000000000 ) ) ;
#9840=CYLINDRICAL_SURFACE ( 'NONE', #5489, 2.000000000000001776 ) ;
#9841=DIRECTION ( 'NONE',  ( -0.000000000000000000, 0.000000000000000000, 1.000000000000000000 ) ) ;
#9844=DIRECTION ( 'NONE',  ( -0.000000000000000000, 1.000000000000000000, -0.000000000000000000 ) ) ;
#9846=EDGE_LOOP ( 'NONE', ( #820, #1438, #6312, #7459, #4465, #1341, #9725, #3244 ) ) ;
#9847=DIRECTION ( 'NONE',  ( -0.000000000000000000, 1.000000000000000000, -0.000000000000000000 ) ) ;
#9849=EDGE_CURVE ( 'NONE', #8972, #4758, #10361, .T. ) ;
#9850=DIRECTION ( 'NONE',  ( 1.000000000000000000, 0.000000000000000000, 0.000000000000000000 ) ) ;
#9852=CARTESIAN_POINT ( 'NONE',  ( -40.00000000000001421, -145.1457019118819005, -44.00000000000001421 ) ) ;
#9853=DIRECTION ( 'NONE',  ( 0.000000000000000000, 0.000000000000000000, -1.000000000000000000 ) ) ;
#9854=DIRECTION ( 'NONE',  ( 1.000000000000000000, 0.000000000000000000, 0.000000000000000000 ) ) ;
#9860=ADVANCED_FACE ( 'NONE', ( #7713 ), #8456, .F. ) ;
#9861=EDGE_LOOP ( 'NONE', ( #976, #3978 ) ) ;
#9863=CARTESIAN_POINT ( 'NONE',  ( 53.40242741783141156, 42.08684478514406635, 25.00000000000000000 ) ) ;
#9867=CARTESIAN_POINT ( 'NONE',  ( -16.29350689640809691, -140.1746510883711778, 27.01918567566963247 ) ) ;
#9868=VECTOR ( 'NONE', #65, 1000.000000000000000 ) ;
#9870=ORIENTED_EDGE ( 'NONE', *, *, #2171, .F. ) ;
#9872=ORIENTED_EDGE ( 'NONE', *, *, #4331, .T. ) ;
#9876=DIRECTION ( 'NONE',  ( 0.000000000000000000, 0.000000000000000000, 1.000000000000000000 ) ) ;
#9878=CARTESIAN_POINT ( 'NONE',  ( 39.99999999999997158, -135.1457019118818721, 39.99999999999997868 ) ) ;
#9881=AXIS2_PLACEMENT_3D ( 'NONE', #1224, #6092, #5245 ) ;
#9883=CARTESIAN_POINT ( 'NONE',  ( -2.293506896408097795, 120.5696653505793705, -20.00000000000000711 ) ) ;
#9884=VERTEX_POINT ( 'NONE', #8352 ) ;
#9886=DIRECTION ( 'NONE',  ( 0.000000000000000000, 1.000000000000000000, 0.000000000000000000 ) ) ;
#9889=CIRCLE ( 'NONE', #2934, 1.999999999999998224 ) ;
#9892=DIRECTION ( 'NONE',  ( -0.000000000000000000, 1.000000000000000000, 0.000000000000000000 ) ) ;
#9894=CARTESIAN_POINT ( 'NONE',  ( -40.00000000000001421, -135.1457019118818721, -40.00000000000002132 ) ) ;
#9897=CARTESIAN_POINT ( 'NONE',  ( 18.34874108452142494, -140.1746510883711778, -97.78965767959371647 ) ) ;
#9899=ORIENTED_EDGE ( 'NONE', *, *, #9379, .T. ) ;
#9902=EDGE_LOOP ( 'NONE', ( #5085, #7653, #6677, #2672 ) ) ;
#9906=DIRECTION ( 'NONE',  ( -1.000000000000000000, 0.000000000000000000, 0.000000000000000000 ) ) ;
#9907=DIRECTION ( 'NONE',  ( 0.000000000000000000, -1.000000000000000000, 0.000000000000000000 ) ) ;
#9908=ORIENTED_EDGE ( 'NONE', *, *, #6715, .T. ) ;
#9914=CIRCLE ( 'NONE', #8548, 3.999999999999996447 ) ;
#9916=DIRECTION ( 'NONE',  ( 1.000000000000000000, -7.780263845122167369E-16, 0.000000000000000000 ) ) ;
#9927=CARTESIAN_POINT ( 'NONE',  ( 4.856471286862176662, 145.0444252872335937, 25.00000000000000000 ) ) ;
#9930=DIRECTION ( 'NONE',  ( 1.000000000000000000, 0.000000000000000000, -0.000000000000000000 ) ) ;
#9932=CARTESIAN_POINT ( 'NONE',  ( -2.293506896408097795, 37.08684478514406635, -25.00000000000000355 ) ) ;
#9934=ORIENTED_EDGE ( 'NONE', *, *, #10252, .F. ) ;
#9936=AXIS2_PLACEMENT_3D ( 'NONE', #6471, #9018, #8915 ) ;
#9937=EDGE_LOOP ( 'NONE', ( #8486, #9017, #2891, #10290, #7650 ) ) ;
#9939=VERTEX_POINT ( 'NONE', #7333 ) ;
#9940=CARTESIAN_POINT ( 'NONE',  ( -40.00000000000002842, -145.1457019118819005, 39.99999999999997868 ) ) ;
#9942=VECTOR ( 'NONE', #6961, 1000.000000000000000 ) ;
#9948=VERTEX_POINT ( 'NONE', #8283 ) ;
#9950=EDGE_CURVE ( 'NONE', #5946, #7078, #6690, .T. ) ;
#9952=ORIENTED_EDGE ( 'NONE', *, *, #7993, .F. ) ;
#9953=LINE ( 'NONE', #6754, #8607 ) ;
#9954=VECTOR ( 'NONE', #10048, 1000.000000000000000 ) ;
#9955=VERTEX_POINT ( 'NONE', #5893 ) ;
#9957=DIRECTION ( 'NONE',  ( 0.000000000000000000, -0.000000000000000000, 1.000000000000000000 ) ) ;
#9958=CARTESIAN_POINT ( 'NONE',  ( 37.23846126345171825, -134.0500961303746692, 25.36885565376192275 ) ) ;
#9959=LINE ( 'NONE', #10104, #3144 ) ;
#9960=DIRECTION ( 'NONE',  ( 0.000000000000000000, 0.000000000000000000, 1.000000000000000000 ) ) ;
#9961=CIRCLE ( 'NONE', #2162, 5.000000000000000888 ) ;
#9965=ADVANCED_FACE ( 'NONE', ( #8175 ), #3462, .F. ) ;
#9966=ORIENTED_EDGE ( 'NONE', *, *, #5833, .F. ) ;
#9972=PLANE ( 'NONE',  #5578 ) ;
#9973=DIRECTION ( 'NONE',  ( -0.000000000000000000, 1.000000000000000000, 0.000000000000000000 ) ) ;
#9974=DIRECTION ( 'NONE',  ( -0.000000000000000000, 1.000000000000000000, -0.000000000000000000 ) ) ;
#9976=DIRECTION ( 'NONE',  ( 0.000000000000000000, 0.000000000000000000, -1.000000000000000000 ) ) ;
#9980=EDGE_CURVE ( 'NONE', #4386, #6270, #5771, .T. ) ;
#9981=( NAMED_UNIT ( * ) SI_UNIT ( $, .STERADIAN. ) SOLID_ANGLE_UNIT ( ) );
#9986=CARTESIAN_POINT ( 'NONE',  ( -25.15769640663940621, -135.1457019118818721, 27.15769640663938489 ) ) ;
#9989=AXIS2_PLACEMENT_3D ( 'NONE', #2020, #8383, #1017 ) ;
#9994=CARTESIAN_POINT ( 'NONE',  ( 37.22759939293836595, -133.1457019118818721, -25.15769640663939910 ) ) ;
#9995=CARTESIAN_POINT ( 'NONE',  ( 0.000000000000000000, -115.1457019118818863, 47.99999999999997868 ) ) ;
#9998=LINE ( 'NONE', #2718, #8681 ) ;
#10003=PLANE ( 'NONE',  #3337 ) ;
#10004=CARTESIAN_POINT ( 'NONE',  ( 37.22797402574886405, -133.4133323156204654, 25.17121823815657677 ) ) ;
#10006=ORIENTED_EDGE ( 'NONE', *, *, #7902, .F. ) ;
#10009=ORIENTED_EDGE ( 'NONE', *, *, #1687, .F. ) ;
#10011=ORIENTED_EDGE ( 'NONE', *, *, #8597, .F. ) ;
#10013=EDGE_CURVE ( 'NONE', #3513, #640, #4151, .T. ) ;
#10014=CARTESIAN_POINT ( 'NONE',  ( -2.293506896408097795, 120.5696653505793705, -20.00000000000000711 ) ) ;
#10015=ADVANCED_FACE ( 'NONE', ( #9026, #7439, #2508, #2712 ), #2615, .F. ) ;
#10017=CARTESIAN_POINT ( 'NONE',  ( -27.15769640663940621, -135.1457019118818721, -3.792811993702496405E-15 ) ) ;
#10019=CARTESIAN_POINT ( 'NONE',  ( -18.34874108452141783, -140.1746510883711778, 29.59847408863694440 ) ) ;
#10021=VECTOR ( 'NONE', #7549, 1000.000000000000000 ) ;
#10022=ORIENTED_EDGE ( 'NONE', *, *, #9396, .T. ) ;
#10025=ADVANCED_FACE ( 'NONE', ( #1343 ), #2076, .T. ) ;
#10029=ORIENTED_EDGE ( 'NONE', *, *, #1293, .F. ) ;
#10033=EDGE_LOOP ( 'NONE', ( #764, #10244, #4530 ) ) ;
#10034=CARTESIAN_POINT ( 'NONE',  ( 37.22759939293836595, -117.1457019118819005, -25.15769640663939910 ) ) ;
#10036=FACE_OUTER_BOUND ( 'NONE', #7597, .T. ) ;
#10037=DIRECTION ( 'NONE',  ( 0.000000000000000000, 0.000000000000000000, -1.000000000000000000 ) ) ;
#10041=DIRECTION ( 'NONE',  ( 0.000000000000000000, 0.7071067811864494290, 0.7071067811866454944 ) ) ;
#10042=EDGE_CURVE ( 'NONE', #8095, #9794, #2871, .T. ) ;
#10044=CIRCLE ( 'NONE', #6999, 19.24539146688411506 ) ;
#10045=DIRECTION ( 'NONE',  ( -1.000000000000000000, 0.000000000000000000, 0.000000000000000000 ) ) ;
#10048=DIRECTION ( 'NONE',  ( 1.396588258780021135E-16, 0.000000000000000000, -1.000000000000000000 ) ) ;
#10049=FACE_OUTER_BOUND ( 'NONE', #6755, .T. ) ;
#10052=ORIENTED_EDGE ( 'NONE', *, *, #3540, .T. ) ;
#10056=EDGE_CURVE ( 'NONE', #10372, #2017, #8547, .T. ) ;
#10057=ORIENTED_EDGE ( 'NONE', *, *, #7804, .T. ) ;
#10059=CIRCLE ( 'NONE', #742, 3.999999999999996447 ) ;
#10061=DIRECTION ( 'NONE',  ( 1.000000000000000000, -9.013708445275205736E-16, 0.000000000000000000 ) ) ;
#10062=CARTESIAN_POINT ( 'NONE',  ( -18.34874108452141783, -140.1746510883711778, -7.212905963064413228 ) ) ;
#10066=CARTESIAN_POINT ( 'NONE',  ( 77.30044127146540234, 73.68369600860394542, 25.00000000000000000 ) ) ;
#10070=EDGE_CURVE ( 'NONE', #3513, #10220, #3075, .T. ) ;
#10071=ORIENTED_EDGE ( 'NONE', *, *, #2681, .F. ) ;
#10076=EDGE_LOOP ( 'NONE', ( #6978, #2068, #5924, #4812 ) ) ;
#10077=FACE_OUTER_BOUND ( 'NONE', #899, .T. ) ;
#10078=SHAPE_REPRESENTATION_RELATIONSHIP ( 'NONE' , 'NONE' ,  #1081, #638 ) ;
#10081=VECTOR ( 'NONE', #2594, 1000.000000000000227 ) ;
#10082=VERTEX_POINT ( 'NONE', #7755 ) ;
#10083=ORIENTED_EDGE ( 'NONE', *, *, #10395, .T. ) ;
#10086=EDGE_CURVE ( 'NONE', #8738, #996, #3677, .T. ) ;
#10091=CYLINDRICAL_SURFACE ( 'NONE', #7560, 5.000000000000001776 ) ;
#10092=DIRECTION ( 'NONE',  ( -1.000000000000000000, 0.000000000000000000, 0.000000000000000000 ) ) ;
#10093=AXIS2_PLACEMENT_3D ( 'NONE', #8976, #2616, #7543 ) ;
#10094=CARTESIAN_POINT ( 'NONE',  ( -2.293506896408097795, 42.08684478514410188, -30.00000000000000355 ) ) ;
#10095=ORIENTED_EDGE ( 'NONE', *, *, #10395, .F. ) ;
#10098=LINE ( 'NONE', #1294, #2014 ) ;
#10099=FACE_OUTER_BOUND ( 'NONE', #9499, .T. ) ;
#10100=AXIS2_PLACEMENT_3D ( 'NONE', #3943, #7126, #9347 ) ;
#10101=EDGE_CURVE ( 'NONE', #5230, #3031, #1883, .T. ) ;
#10102=DIRECTION ( 'NONE',  ( 0.000000000000000000, 1.000000000000000000, 0.000000000000000000 ) ) ;
#10103=CARTESIAN_POINT ( 'NONE',  ( 14.70649310359190309, 80.56966535057935630, -20.00000000000000711 ) ) ;
#10104=CARTESIAN_POINT ( 'NONE',  ( 32.59878849545336976, 32.08684478514406635, 30.00000000000000355 ) ) ;
#10116=AXIS2_PLACEMENT_3D ( 'NONE', #8869, #1557, #7924 ) ;
#10121=CARTESIAN_POINT ( 'NONE',  ( 37.71464122736488633, -135.1457019118818721, 27.15769640663938489 ) ) ;
#10123=CARTESIAN_POINT ( 'NONE',  ( -23.15769640663940976, -117.1457019118819005, 27.15769640663938489 ) ) ;
#10128=ORIENTED_EDGE ( 'NONE', *, *, #7336, .T. ) ;
#10130=ORIENTED_EDGE ( 'NONE', *, *, #1656, .F. ) ;
#10131=DIRECTION ( 'NONE',  ( -0.000000000000000000, 1.000000000000000000, -0.000000000000000000 ) ) ;
#10132=( NAMED_UNIT ( * ) PLANE_ANGLE_UNIT ( ) SI_UNIT ( $, .RADIAN. ) );
#10135=EDGE_CURVE ( 'NONE', #4046, #7873, #391, .T. ) ;
#10139=ORIENTED_EDGE ( 'NONE', *, *, #757, .F. ) ;
#10142=DIRECTION ( 'NONE',  ( 6.982941293900105430E-16, -0.000000000000000000, -1.000000000000000000 ) ) ;
#10145=EDGE_CURVE ( 'NONE', #426, #4585, #9292, .T. ) ;
#10148=CARTESIAN_POINT ( 'NONE',  ( 32.59878849545336976, 32.08684478514406635, -12.49999999999999289 ) ) ;
#10153=ORIENTED_EDGE ( 'NONE', *, *, #1188, .T. ) ;
#10157=DIRECTION ( 'NONE',  ( -1.000000000000000000, 0.000000000000000000, -9.776117811460135374E-16 ) ) ;
#10161=DIRECTION ( 'NONE',  ( 0.000000000000000000, -1.000000000000000000, 0.000000000000000000 ) ) ;
#10165=PLANE ( 'NONE',  #7392 ) ;
#10168=CYLINDRICAL_SURFACE ( 'NONE', #9765, 10.00000000000000178 ) ;
#10172=DIRECTION ( 'NONE',  ( 0.000000000000000000, 1.000000000000000000, -0.000000000000000000 ) ) ;
#10173=CARTESIAN_POINT ( 'NONE',  ( -16.29350689640809691, -140.1746510883711778, 23.72119897386845722 ) ) ;
#10177=ORIENTED_EDGE ( 'NONE', *, *, #5334, .T. ) ;
#10179=CIRCLE ( 'NONE', #2889, 5.000000000000000888 ) ;
#10180=ORIENTED_EDGE ( 'NONE', *, *, #7467, .F. ) ;
#10181=DIRECTION ( 'NONE',  ( 1.734723475976805319E-15, -0.000000000000000000, -1.000000000000000000 ) ) ;
#10182=FACE_OUTER_BOUND ( 'NONE', #9861, .T. ) ;
#10186=AXIS2_PLACEMENT_3D ( 'NONE', #7491, #7383, #1285 ) ;
#10188=ORIENTED_EDGE ( 'NONE', *, *, #6063, .F. ) ;
#10190=AXIS2_PLACEMENT_3D ( 'NONE', #2987, #4627, #3879 ) ;
#10192=CIRCLE ( 'NONE', #874, 1.999999999999998224 ) ;
#10193=EDGE_LOOP ( 'NONE', ( #3897, #10272, #58, #8271 ) ) ;
#10195=DIRECTION ( 'NONE',  ( 0.000000000000000000, 0.000000000000000000, -1.000000000000000000 ) ) ;
#10197=LINE ( 'NONE', #8762, #4341 ) ;
#10198=AXIS2_PLACEMENT_3D ( 'NONE', #9078, #1024, #5895 ) ;
#10199=ORIENTED_EDGE ( 'NONE', *, *, #251, .F. ) ;
#10202=EDGE_CURVE ( 'NONE', #898, #10372, #1553, .T. ) ;
#10204=EDGE_CURVE ( 'NONE', #5617, #59, #7972, .T. ) ;
#10206=DIRECTION ( 'NONE',  ( -0.000000000000000000, -0.000000000000000000, -1.000000000000000000 ) ) ;
#10208=CIRCLE ( 'NONE', #2754, 2.000000000000001776 ) ;
#10209=DIRECTION ( 'NONE',  ( 1.000000000000000000, 0.000000000000000000, -0.000000000000000000 ) ) ;
#10210=DIRECTION ( 'NONE',  ( 0.000000000000000000, 0.000000000000000000, 1.000000000000000000 ) ) ;
#10213=FACE_OUTER_BOUND ( 'NONE', #3164, .T. ) ;
#10218=EDGE_CURVE ( 'NONE', #7105, #6373, #2241, .T. ) ;
#10219=DIRECTION ( 'NONE',  ( -0.000000000000000000, 1.000000000000000000, 0.000000000000000000 ) ) ;
#10220=VERTEX_POINT ( 'NONE', #2344 ) ;
#10221=VERTEX_POINT ( 'NONE', #10402 ) ;
#10222=B_SPLINE_CURVE_WITH_KNOTS ( 'NONE', 3,
 ( #3477, #3635, #10004, #2037, #2834, #9958, #5265, #5222, #8504, #8349, #8454, #7711, #1143, #1884, #6066, #2778 ),
 .UNSPECIFIED., .F., .F.,
 ( 4, 2, 2, 2, 2, 2, 2, 4 ),
 ( 0.000000000000000000, 0.0003991717881400778088, 0.0007983435762801556175, 0.001197515364420233481, 0.001596687152560311235, 0.002395030728840411450, 0.002794202516980451908, 0.003193374305120491932 ),
 .UNSPECIFIED. ) ;
#10224=CARTESIAN_POINT ( 'NONE',  ( 27.15769640663936713, -133.1457019118818721, 27.15769640663938489 ) ) ;
#10226=CARTESIAN_POINT ( 'NONE',  ( 33.55285093437175448, 29.14909237014566301, 12.50000000000000000 ) ) ;
#10230=DIRECTION ( 'NONE',  ( 1.387778780781445676E-16, -0.000000000000000000, -1.000000000000000000 ) ) ;
#10231=ORIENTED_EDGE ( 'NONE', *, *, #429, .F. ) ;
#10232=CIRCLE ( 'NONE', #4969, 4.000000000000000000 ) ;
#10235=VERTEX_POINT ( 'NONE', #7123 ) ;
#10236=DIRECTION ( 'NONE',  ( -1.000000000000000000, 0.000000000000000000, 0.000000000000000000 ) ) ;
#10238=CARTESIAN_POINT ( 'NONE',  ( -50.00000000000002842, -135.1457019118818721, 26.62179802177713484 ) ) ;
#10244=ORIENTED_EDGE ( 'NONE', *, *, #9365, .T. ) ;
#10245=ORIENTED_EDGE ( 'NONE', *, *, #5786, .F. ) ;
#10248=DIRECTION ( 'NONE',  ( 0.000000000000000000, 1.000000000000000000, -0.000000000000000000 ) ) ;
#10251=CARTESIAN_POINT ( 'NONE',  ( 73.53765631853929108, 70.39106037767955115, 25.00000000000000000 ) ) ;
#10252=EDGE_CURVE ( 'NONE', #3180, #2069, #6368, .T. ) ;
#10260=CARTESIAN_POINT ( 'NONE',  ( 4.856471286862176662, 145.0444252872335937, 30.00000000000000355 ) ) ;
#10261=ADVANCED_FACE ( 'NONE', ( #8856 ), #5947, .F. ) ;
#10270=TOROIDAL_SURFACE ( 'NONE', #3672, 24.24539146688411506, 5.000000000000000000 ) ;
#10272=ORIENTED_EDGE ( 'NONE', *, *, #4375, .F. ) ;
#10274=CARTESIAN_POINT ( 'NONE',  ( -48.00000000000002132, -115.1457019118818863, 23.15769640663938134 ) ) ;
#10276=EDGE_LOOP ( 'NONE', ( #6901, #7808, #8921, #10052 ) ) ;
#10278=DIRECTION ( 'NONE',  ( -1.000000000000000000, 0.000000000000000000, 0.000000000000000000 ) ) ;
#10279=EDGE_CURVE ( 'NONE', #10221, #8048, #10192, .T. ) ;
#10280=EDGE_CURVE ( 'NONE', #36, #2136, #206, .T. ) ;
#10284=DIRECTION ( 'NONE',  ( 1.734723475976806848E-16, 0.000000000000000000, 1.000000000000000000 ) ) ;
#10289=VECTOR ( 'NONE', #1934, 1000.000000000000000 ) ;
#10290=ORIENTED_EDGE ( 'NONE', *, *, #9363, .F. ) ;
#10291=DIRECTION ( 'NONE',  ( -0.000000000000000000, 1.000000000000000000, -0.000000000000000000 ) ) ;
#10292=DIRECTION ( 'NONE',  ( 0.000000000000000000, 0.000000000000000000, -1.000000000000000000 ) ) ;
#10297=VECTOR ( 'NONE', #5732, 1000.000000000000000 ) ;
#10298=EDGE_CURVE ( 'NONE', #2542, #3031, #6266, .T. ) ;
#10301=ORIENTED_EDGE ( 'NONE', *, *, #2415, .T. ) ;
#10303=EDGE_CURVE ( 'NONE', #3453, #8369, #4192, .T. ) ;
#10305=ORIENTED_EDGE ( 'NONE', *, *, #1799, .T. ) ;
#10306=EDGE_LOOP ( 'NONE', ( #824, #3120, #2092, #4301 ) ) ;
#10307=DIRECTION ( 'NONE',  ( -0.000000000000000000, -0.000000000000000000, -1.000000000000000000 ) ) ;
#10309=DIRECTION ( 'NONE',  ( 0.6585271261848805180, -0.7525569905852198538, 0.000000000000000000 ) ) ;
#10311=CARTESIAN_POINT ( 'NONE',  ( 39.99999999999998579, -135.1457019118818721, -44.00000000000001421 ) ) ;
#10314=VECTOR ( 'NONE', #5487, 1000.000000000000000 ) ;
#10317=PLANE ( 'NONE',  #2155 ) ;
#10320=DIRECTION ( 'NONE',  ( 1.387778780781445676E-16, 0.000000000000000000, -1.000000000000000000 ) ) ;
#10329=ORIENTED_EDGE ( 'NONE', *, *, #5397, .T. ) ;
#10331=CARTESIAN_POINT ( 'NONE',  ( 23.15769640663936713, -115.1457019118818863, 47.99999999999997868 ) ) ;
#10333=DIRECTION ( 'NONE',  ( 1.000000000000000000, 0.000000000000000000, -0.000000000000000000 ) ) ;
#10335=DIRECTION ( 'NONE',  ( 1.000000000000000000, 0.000000000000000000, 0.000000000000000000 ) ) ;
#10338=CARTESIAN_POINT ( 'NONE',  ( 42.22511195853869026, -135.1457019118818721, -30.00000000000000355 ) ) ;
#10341=ADVANCED_FACE ( 'NONE', ( #3290 ), #2907, .T. ) ;
#10342=ORIENTED_EDGE ( 'NONE', *, *, #8857, .T. ) ;
#10343=DIRECTION ( 'NONE',  ( 1.000000000000000000, 3.469446951953610639E-15, -0.000000000000000000 ) ) ;
#10349=ORIENTED_EDGE ( 'NONE', *, *, #8317, .F. ) ;
#10350=EDGE_LOOP ( 'NONE', ( #9561, #219, #5812, #301, #3887, #4034, #7013, #10011 ) ) ;
#10351=ADVANCED_FACE ( 'NONE', ( #2600 ), #2396, .F. ) ;
#10353=CARTESIAN_POINT ( 'NONE',  ( -50.00000000000001421, -134.3099331815685389, -24.41868145091762798 ) ) ;
#10354=CIRCLE ( 'NONE', #8649, 3.297986701801175258 ) ;
#10360=AXIS2_PLACEMENT_3D ( 'NONE', #1349, #4730, #705 ) ;
#10361=CIRCLE ( 'NONE', #7983, 10.00000000000000178 ) ;
#10362=EDGE_LOOP ( 'NONE', ( #10199, #9312, #9872, #3371 ) ) ;
#10366=DIRECTION ( 'NONE',  ( -0.000000000000000000, -0.000000000000000000, -1.000000000000000000 ) ) ;
#10367=EDGE_CURVE ( 'NONE', #3381, #7949, #8826, .T. ) ;
#10369=ORIENTED_EDGE ( 'NONE', *, *, #655, .F. ) ;
#10370=CARTESIAN_POINT ( 'NONE',  ( 73.53765631853929108, 70.39106037767953694, -30.00000000000000355 ) ) ;
#10372=VERTEX_POINT ( 'NONE', #6679 ) ;
#10374=CARTESIAN_POINT ( 'NONE',  ( -40.00000000000001421, -135.1457019118818721, -40.00000000000002132 ) ) ;
#10384=CARTESIAN_POINT ( 'NONE',  ( -48.00000000000002132, -117.1457019118819005, -23.15769640663945594 ) ) ;
#10385=EDGE_CURVE ( 'NONE', #3749, #7484, #4262, .T. ) ;
#10386=CIRCLE ( 'NONE', #2593, 4.025000000000000355 ) ;
#10387=ORIENTED_EDGE ( 'NONE', *, *, #8967, .F. ) ;
#10388=CARTESIAN_POINT ( 'NONE',  ( 39.99999999999998579, -145.1457019118819005, -40.00000000000002132 ) ) ;
#10389=EDGE_LOOP ( 'NONE', ( #569, #3201, #6983, #8998, #319, #8545, #10006, #6152, #3332, #1014 ) ) ;
#10392=DIRECTION ( 'NONE',  ( 0.000000000000000000, -1.000000000000000000, 0.000000000000000000 ) ) ;
#10394=EDGE_LOOP ( 'NONE', ( #4669, #754, #1778, #6452, #3307, #982, #5385 ) ) ;
#10395=EDGE_CURVE ( 'NONE', #7038, #8587, #3423, .T. ) ;
#10396=TOROIDAL_SURFACE ( 'NONE', #4125, 4.000000000000000000, 2.000000000000000000 ) ;
#10398=EDGE_CURVE ( 'NONE', #5542, #991, #267, .T. ) ;
#10400=EDGE_LOOP ( 'NONE', ( #8130, #6095, #7780, #5809 ) ) ;
#10401=CARTESIAN_POINT ( 'NONE',  ( -50.00000000000001421, -135.0799163051958942, -25.93999053166059099 ) ) ;
#10402=CARTESIAN_POINT ( 'NONE',  ( -25.15769640663939199, -117.1457019118819005, -27.15769640663944173 ) ) ;
#10406=CARTESIAN_POINT ( 'NONE',  ( 39.99999999999998579, -115.1457019118818863, -40.00000000000002132 ) ) ;
#10409=ORIENTED_EDGE ( 'NONE', *, *, #1581, .T. ) ;
#10411=AXIS2_PLACEMENT_3D ( 'NONE', #10469, #8871, #1561 ) ;
#10412=ORIENTED_EDGE ( 'NONE', *, *, #9980, .F. ) ;
#10415=CARTESIAN_POINT ( 'NONE',  ( -16.29350689640809691, -186.9457019118818835, -27.01918567566963247 ) ) ;
#10416=CARTESIAN_POINT ( 'NONE',  ( 37.22759939293836595, -116.8755810935459323, 25.15769640663938489 ) ) ;
#10420=CARTESIAN_POINT ( 'NONE',  ( -40.00000000000002842, -135.1707019118818778, 39.99999999999997868 ) ) ;
#10422=ORIENTED_EDGE ( 'NONE', *, *, #128, .T. ) ;
#10426=VECTOR ( 'NONE', #7712, 1000.000000000000000 ) ;
#10431=DIRECTION ( 'NONE',  ( 1.396588258780021135E-16, 0.000000000000000000, -1.000000000000000000 ) ) ;
#10439=VECTOR ( 'NONE', #9455, 1000.000000000000000 ) ;
#10441=DIRECTION ( 'NONE',  ( 0.000000000000000000, 0.000000000000000000, 1.000000000000000000 ) ) ;
#10443=AXIS2_PLACEMENT_3D ( 'NONE', #5601, #5554, #683 ) ;
#10446=DIRECTION ( 'NONE',  ( 0.000000000000000000, 0.000000000000000000, 1.000000000000000000 ) ) ;
#10448=AXIS2_PLACEMENT_3D ( 'NONE', #568, #6981, #3803 ) ;
#10449=ORIENTED_EDGE ( 'NONE', *, *, #5667, .T. ) ;
#10450=ORIENTED_EDGE ( 'NONE', *, *, #9442, .F. ) ;
#10451=ORIENTED_EDGE ( 'NONE', *, *, #6119, .F. ) ;
#10452=ADVANCED_FACE ( 'NONE', ( #2913 ), #1221, .T. ) ;
#10453=CARTESIAN_POINT ( 'NONE',  ( -50.00000000000001421, -135.1457019118818721, -26.27514770175552528 ) ) ;
#10454=DIRECTION ( 'NONE',  ( 0.000000000000000000, 0.000000000000000000, -1.000000000000000000 ) ) ;
#10455=AXIS2_PLACEMENT_3D ( 'NONE', #7490, #5837, #4205 ) ;
#10456=CARTESIAN_POINT ( 'NONE',  ( -48.00000000000002132, -115.1457019118818863, -23.15769640663945594 ) ) ;
#10458=AXIS2_PLACEMENT_3D ( 'NONE', #5405, #6896, #1277 ) ;
#10459=CARTESIAN_POINT ( 'NONE',  ( 80.08610854271792334, 54.73418909528891874, 25.00000000000000000 ) ) ;
#10467=ADVANCED_FACE ( 'NONE', ( #10182 ), #9169, .T. ) ;
#10468=CIRCLE ( 'NONE', #7418, 4.000000000000000000 ) ;
#10469=CARTESIAN_POINT ( 'NONE',  ( -16.29350689640809691, -115.1457019118818863, -27.01918567566963247 ) ) ;
#10472=DIRECTION ( 'NONE',  ( 0.000000000000000000, -1.000000000000000000, 0.000000000000000000 ) ) ;
#10476=EDGE_LOOP ( 'NONE', ( #5483, #3253, #4175, #9024, #1827, #232 ) ) ;
#10491=COLOUR_RGB('Dark Blue',0.08,0.2,0.34);
#10492=FILL_AREA_STYLE_COLOUR('',#10491);
#10493=FILL_AREA_STYLE('',(#10492));
#10494=SURFACE_STYLE_FILL_AREA(#10493);
#10495=SURFACE_SIDE_STYLE('',(#10494));
#10496=SURFACE_STYLE_USAGE(.BOTH.,#10495);
#10497=PRESENTATION_STYLE_ASSIGNMENT((#10496));
ENDSEC;
END-ISO-10303-21;
